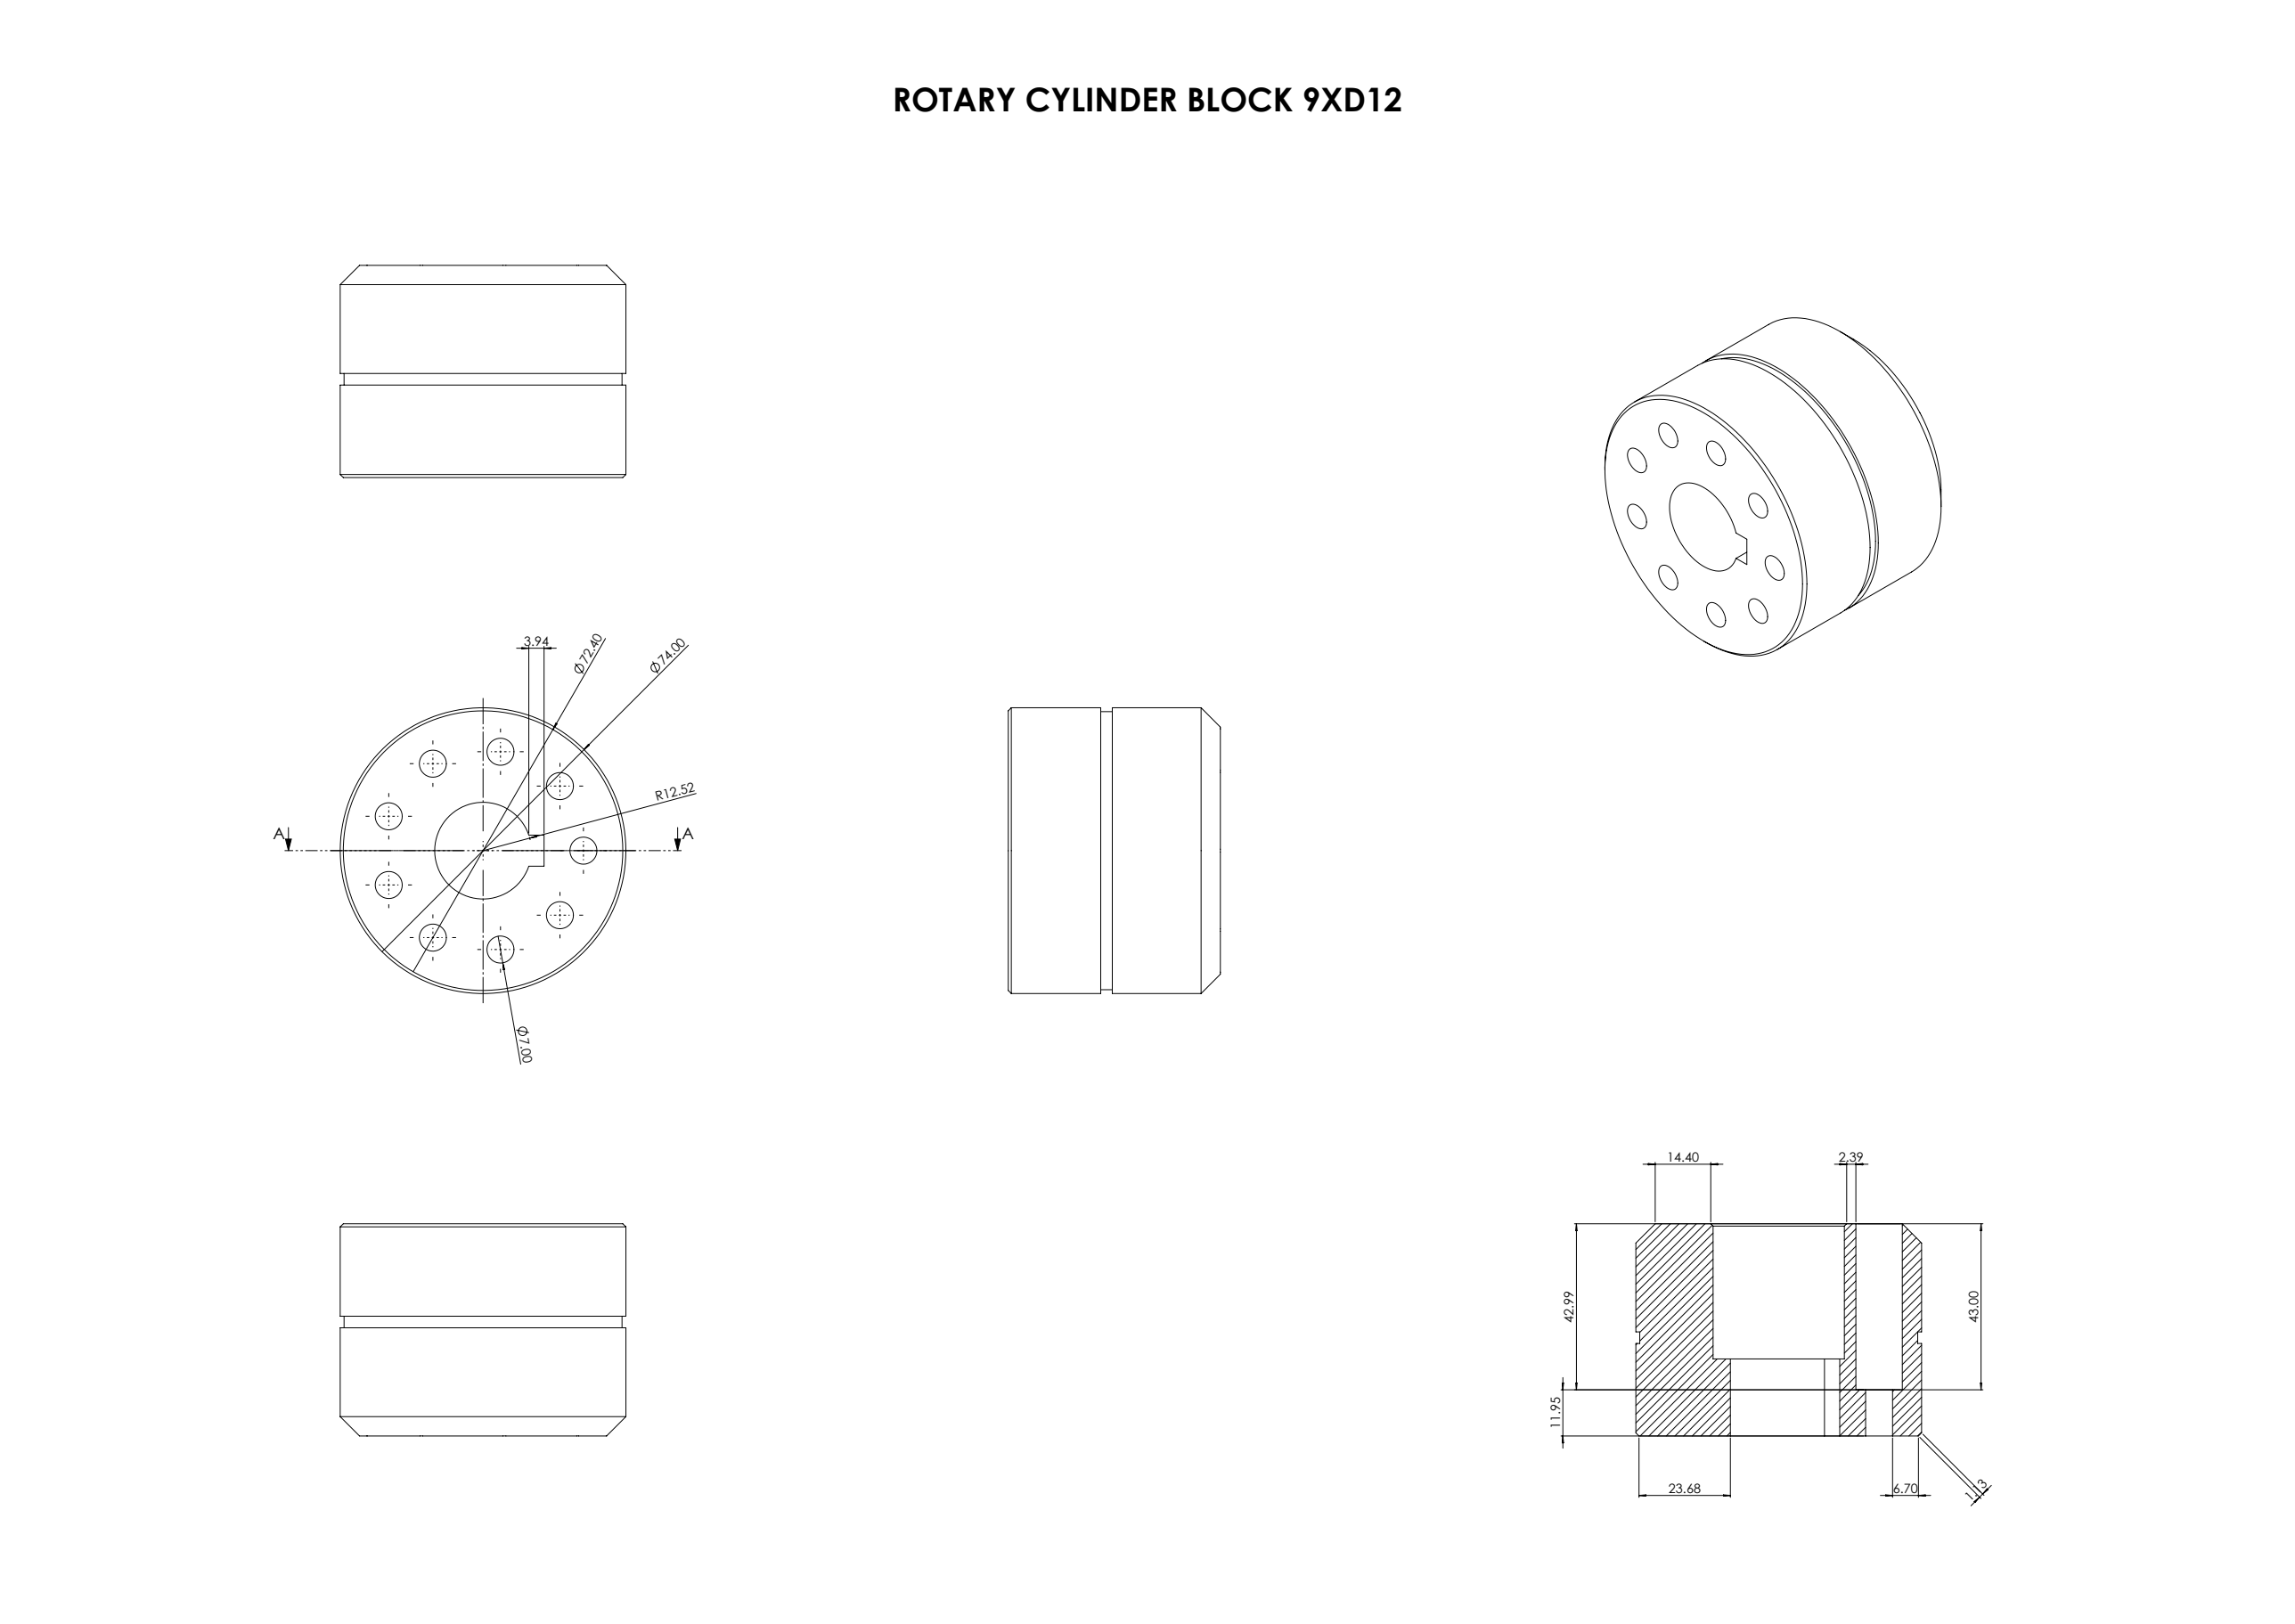
ISO-10303-21;
HEADER;
/* Generated by software containing ST-Developer
 * from STEP Tools, Inc. (www.steptools.com) 
 */

FILE_DESCRIPTION(
/* description */ (''),
/* implementation_level */ '2;1');

FILE_NAME(
/* name */ '05_Rotary_Cylinder_Block_9xD12.step',
/* time_stamp */ '2026-10-23T00:52:27+05:00',
/* author */ (''),
/* organization */ (''),
/* preprocessor_version */ 'ST-DEVELOPER v20.2',
/* originating_system */ 'Autodesk Translation Framework v15.15.0.0',
/* authorisation */ '');

FILE_SCHEMA (('AUTOMOTIVE_DESIGN { 1 0 10303 214 3 1 1 }'));
ENDSEC;

DATA;
#10=MECHANICAL_DESIGN_GEOMETRIC_PRESENTATION_REPRESENTATION('',(#1557),#59204);
#683=B_SPLINE_CURVE_WITH_KNOTS('',3,(#42129,#42130,#42131,#42132,#42133,
#42134),.UNSPECIFIED.,.F.,.F.,(4,2,4),(1.68069680516896,1.71912851411125,
1.75756022305355),.UNSPECIFIED.);
#684=B_SPLINE_CURVE_WITH_KNOTS('',3,(#42145,#42146,#42147,#42148,#42149,
#42150),.UNSPECIFIED.,.F.,.F.,(4,2,4),(1.68069680516896,1.71912851411125,
1.75756022305355),.UNSPECIFIED.);
#685=B_SPLINE_CURVE_WITH_KNOTS('',3,(#42161,#42162,#42163,#42164,#42165,
#42166),.UNSPECIFIED.,.F.,.F.,(4,2,4),(1.68069680516896,1.71912851411125,
1.75756022305355),.UNSPECIFIED.);
#686=B_SPLINE_CURVE_WITH_KNOTS('',3,(#42177,#42178,#42179,#42180,#42181,
#42182),.UNSPECIFIED.,.F.,.F.,(4,2,4),(1.68069680516896,1.71912851411125,
1.75756022305355),.UNSPECIFIED.);
#687=B_SPLINE_CURVE_WITH_KNOTS('',3,(#42193,#42194,#42195,#42196,#42197,
#42198),.UNSPECIFIED.,.F.,.F.,(4,2,4),(1.68069680516897,1.71912851411125,
1.75756022305354),.UNSPECIFIED.);
#688=B_SPLINE_CURVE_WITH_KNOTS('',3,(#42209,#42210,#42211,#42212,#42213,
#42214),.UNSPECIFIED.,.F.,.F.,(4,2,4),(1.68069680516896,1.71912851411125,
1.75756022305355),.UNSPECIFIED.);
#689=B_SPLINE_CURVE_WITH_KNOTS('',3,(#42225,#42226,#42227,#42228,#42229,
#42230),.UNSPECIFIED.,.F.,.F.,(4,2,4),(1.68069680516896,1.71912851411125,
1.75756022305355),.UNSPECIFIED.);
#690=B_SPLINE_CURVE_WITH_KNOTS('',3,(#42241,#42242,#42243,#42244,#42245,
#42246),.UNSPECIFIED.,.F.,.F.,(4,2,4),(1.68069680516896,1.71912851411125,
1.75756022305355),.UNSPECIFIED.);
#691=B_SPLINE_CURVE_WITH_KNOTS('',3,(#42257,#42258,#42259,#42260,#42261,
#42262),.UNSPECIFIED.,.F.,.F.,(4,2,4),(1.68069680516896,1.71912851411125,
1.75756022305355),.UNSPECIFIED.);
#1517=SHAPE_REPRESENTATION_RELATIONSHIP('SRR','None',#59306,#1537);
#1537=ADVANCED_BREP_SHAPE_REPRESENTATION('',(#1584),#59193);
#1557=STYLED_ITEM('',(#59565),#1584);
#1584=MANIFOLD_SOLID_BREP('Cylinder block',#22813);
#1647=FACE_BOUND('',#4356,.T.);
#1648=FACE_BOUND('',#4359,.T.);
#1649=FACE_BOUND('',#4365,.T.);
#1650=FACE_BOUND('',#4377,.T.);
#1651=FACE_BOUND('',#4380,.T.);
#1652=FACE_BOUND('',#4383,.T.);
#1653=FACE_BOUND('',#4386,.T.);
#1654=FACE_BOUND('',#4389,.T.);
#1655=FACE_BOUND('',#4392,.T.);
#1656=FACE_BOUND('',#4395,.T.);
#1657=FACE_BOUND('',#4398,.T.);
#1658=FACE_BOUND('',#4401,.T.);
#1659=FACE_BOUND('',#4403,.T.);
#1660=FACE_BOUND('',#4410,.T.);
#1661=FACE_BOUND('',#4411,.T.);
#1662=FACE_BOUND('',#4412,.T.);
#1663=FACE_BOUND('',#4413,.T.);
#1664=FACE_BOUND('',#4414,.T.);
#1665=FACE_BOUND('',#4415,.T.);
#1666=FACE_BOUND('',#4416,.T.);
#1667=FACE_BOUND('',#4417,.T.);
#1668=FACE_BOUND('',#4418,.T.);
#1669=FACE_BOUND('',#4419,.T.);
#2003=PLANE('',#23610);
#2004=PLANE('',#23615);
#2005=PLANE('',#23619);
#2006=PLANE('',#23620);
#2007=PLANE('',#23621);
#2008=PLANE('',#23622);
#2009=PLANE('',#23656);
#2010=PLANE('',#23661);
#2011=PLANE('',#23666);
#2012=PLANE('',#23671);
#2013=PLANE('',#23676);
#2014=PLANE('',#23681);
#2015=PLANE('',#23686);
#2016=PLANE('',#23691);
#2017=PLANE('',#23696);
#2018=PLANE('',#23697);
#2019=PLANE('',#23717);
#2481=CYLINDRICAL_SURFACE('',#23613,3.6);
#2482=CYLINDRICAL_SURFACE('',#23617,3.7);
#2483=CYLINDRICAL_SURFACE('',#23625,0.35);
#2484=CYLINDRICAL_SURFACE('',#23628,0.35);
#2485=CYLINDRICAL_SURFACE('',#23631,0.35);
#2486=CYLINDRICAL_SURFACE('',#23634,0.35);
#2487=CYLINDRICAL_SURFACE('',#23637,0.35);
#2488=CYLINDRICAL_SURFACE('',#23640,0.35);
#2489=CYLINDRICAL_SURFACE('',#23643,0.35);
#2490=CYLINDRICAL_SURFACE('',#23646,0.35);
#2491=CYLINDRICAL_SURFACE('',#23649,0.35);
#2492=CYLINDRICAL_SURFACE('',#23652,0.601);
#2493=CYLINDRICAL_SURFACE('',#23657,0.601);
#2494=CYLINDRICAL_SURFACE('',#23662,0.601);
#2495=CYLINDRICAL_SURFACE('',#23667,0.601);
#2496=CYLINDRICAL_SURFACE('',#23672,0.601);
#2497=CYLINDRICAL_SURFACE('',#23677,0.601);
#2498=CYLINDRICAL_SURFACE('',#23682,0.601);
#2499=CYLINDRICAL_SURFACE('',#23687,0.601);
#2500=CYLINDRICAL_SURFACE('',#23692,0.601);
#2501=CYLINDRICAL_SURFACE('',#23709,1.7);
#2502=CYLINDRICAL_SURFACE('',#23713,3.7);
#2503=CYLINDRICAL_SURFACE('',#23719,1.252);
#3002=FACE_OUTER_BOUND('',#4355,.T.);
#3003=FACE_OUTER_BOUND('',#4357,.T.);
#3004=FACE_OUTER_BOUND('',#4358,.T.);
#3005=FACE_OUTER_BOUND('',#4360,.T.);
#3006=FACE_OUTER_BOUND('',#4361,.T.);
#3007=FACE_OUTER_BOUND('',#4362,.T.);
#3008=FACE_OUTER_BOUND('',#4363,.T.);
#3009=FACE_OUTER_BOUND('',#4364,.T.);
#3010=FACE_OUTER_BOUND('',#4366,.T.);
#3011=FACE_OUTER_BOUND('',#4367,.T.);
#3012=FACE_OUTER_BOUND('',#4368,.T.);
#3013=FACE_OUTER_BOUND('',#4369,.T.);
#3014=FACE_OUTER_BOUND('',#4370,.T.);
#3015=FACE_OUTER_BOUND('',#4371,.T.);
#3016=FACE_OUTER_BOUND('',#4372,.T.);
#3017=FACE_OUTER_BOUND('',#4373,.T.);
#3018=FACE_OUTER_BOUND('',#4374,.T.);
#3019=FACE_OUTER_BOUND('',#4375,.T.);
#3020=FACE_OUTER_BOUND('',#4376,.T.);
#3021=FACE_OUTER_BOUND('',#4378,.T.);
#3022=FACE_OUTER_BOUND('',#4379,.T.);
#3023=FACE_OUTER_BOUND('',#4381,.T.);
#3024=FACE_OUTER_BOUND('',#4382,.T.);
#3025=FACE_OUTER_BOUND('',#4384,.T.);
#3026=FACE_OUTER_BOUND('',#4385,.T.);
#3027=FACE_OUTER_BOUND('',#4387,.T.);
#3028=FACE_OUTER_BOUND('',#4388,.T.);
#3029=FACE_OUTER_BOUND('',#4390,.T.);
#3030=FACE_OUTER_BOUND('',#4391,.T.);
#3031=FACE_OUTER_BOUND('',#4393,.T.);
#3032=FACE_OUTER_BOUND('',#4394,.T.);
#3033=FACE_OUTER_BOUND('',#4396,.T.);
#3034=FACE_OUTER_BOUND('',#4397,.T.);
#3035=FACE_OUTER_BOUND('',#4399,.T.);
#3036=FACE_OUTER_BOUND('',#4400,.T.);
#3037=FACE_OUTER_BOUND('',#4402,.T.);
#3038=FACE_OUTER_BOUND('',#4404,.T.);
#3039=FACE_OUTER_BOUND('',#4405,.T.);
#3040=FACE_OUTER_BOUND('',#4406,.T.);
#3041=FACE_OUTER_BOUND('',#4407,.T.);
#3042=FACE_OUTER_BOUND('',#4408,.T.);
#3043=FACE_OUTER_BOUND('',#4409,.T.);
#3044=FACE_OUTER_BOUND('',#4420,.T.);
#4355=EDGE_LOOP('',(#16216));
#4356=EDGE_LOOP('',(#16217));
#4357=EDGE_LOOP('',(#16218,#16219,#16220,#16221));
#4358=EDGE_LOOP('',(#16222));
#4359=EDGE_LOOP('',(#16223));
#4360=EDGE_LOOP('',(#16224,#16225,#16226,#16227));
#4361=EDGE_LOOP('',(#16228,#16229,#16230,#16231));
#4362=EDGE_LOOP('',(#16232,#16233,#16234,#16235));
#4363=EDGE_LOOP('',(#16236,#16237,#16238,#16239));
#4364=EDGE_LOOP('',(#16240));
#4365=EDGE_LOOP('',(#16241,#16242,#16243,#16244));
#4366=EDGE_LOOP('',(#16245,#16246,#16247,#16248));
#4367=EDGE_LOOP('',(#16249,#16250,#16251,#16252));
#4368=EDGE_LOOP('',(#16253,#16254,#16255,#16256));
#4369=EDGE_LOOP('',(#16257,#16258,#16259,#16260));
#4370=EDGE_LOOP('',(#16261,#16262,#16263,#16264));
#4371=EDGE_LOOP('',(#16265,#16266,#16267,#16268));
#4372=EDGE_LOOP('',(#16269,#16270,#16271,#16272));
#4373=EDGE_LOOP('',(#16273,#16274,#16275,#16276));
#4374=EDGE_LOOP('',(#16277,#16278,#16279,#16280));
#4375=EDGE_LOOP('',(#16281,#16282,#16283,#16284,#16285,#16286));
#4376=EDGE_LOOP('',(#16287));
#4377=EDGE_LOOP('',(#16288));
#4378=EDGE_LOOP('',(#16289,#16290,#16291,#16292,#16293,#16294));
#4379=EDGE_LOOP('',(#16295));
#4380=EDGE_LOOP('',(#16296));
#4381=EDGE_LOOP('',(#16297,#16298,#16299,#16300,#16301,#16302));
#4382=EDGE_LOOP('',(#16303));
#4383=EDGE_LOOP('',(#16304));
#4384=EDGE_LOOP('',(#16305,#16306,#16307,#16308,#16309,#16310));
#4385=EDGE_LOOP('',(#16311));
#4386=EDGE_LOOP('',(#16312));
#4387=EDGE_LOOP('',(#16313,#16314,#16315,#16316,#16317,#16318));
#4388=EDGE_LOOP('',(#16319));
#4389=EDGE_LOOP('',(#16320));
#4390=EDGE_LOOP('',(#16321,#16322,#16323,#16324,#16325,#16326));
#4391=EDGE_LOOP('',(#16327));
#4392=EDGE_LOOP('',(#16328));
#4393=EDGE_LOOP('',(#16329,#16330,#16331,#16332,#16333,#16334));
#4394=EDGE_LOOP('',(#16335));
#4395=EDGE_LOOP('',(#16336));
#4396=EDGE_LOOP('',(#16337,#16338,#16339,#16340,#16341,#16342));
#4397=EDGE_LOOP('',(#16343));
#4398=EDGE_LOOP('',(#16344));
#4399=EDGE_LOOP('',(#16345,#16346,#16347,#16348,#16349,#16350));
#4400=EDGE_LOOP('',(#16351));
#4401=EDGE_LOOP('',(#16352));
#4402=EDGE_LOOP('',(#16353,#16354,#16355,#16356,#16357,#16358,#16359,#16360,
#16361,#16362,#16363,#16364,#16365,#16366,#16367,#16368,#16369,#16370,#16371,
#16372,#16373,#16374,#16375,#16376,#16377,#16378,#16379,#16380));
#4403=EDGE_LOOP('',(#16381));
#4404=EDGE_LOOP('',(#16382,#16383,#16384,#16385));
#4405=EDGE_LOOP('',(#16386,#16387,#16388,#16389));
#4406=EDGE_LOOP('',(#16390,#16391,#16392,#16393,#16394,#16395,#16396,#16397,
#16398,#16399,#16400,#16401,#16402,#16403,#16404,#16405,#16406,#16407,#16408,
#16409,#16410,#16411));
#4407=EDGE_LOOP('',(#16412,#16413,#16414,#16415));
#4408=EDGE_LOOP('',(#16416,#16417,#16418,#16419));
#4409=EDGE_LOOP('',(#16420));
#4410=EDGE_LOOP('',(#16421));
#4411=EDGE_LOOP('',(#16422));
#4412=EDGE_LOOP('',(#16423));
#4413=EDGE_LOOP('',(#16424));
#4414=EDGE_LOOP('',(#16425));
#4415=EDGE_LOOP('',(#16426));
#4416=EDGE_LOOP('',(#16427));
#4417=EDGE_LOOP('',(#16428));
#4418=EDGE_LOOP('',(#16429));
#4419=EDGE_LOOP('',(#16430,#16431,#16432,#16433));
#4420=EDGE_LOOP('',(#16434,#16435,#16436,#16437));
#5884=LINE('',#42039,#7317);
#5885=LINE('',#42045,#7318);
#5886=LINE('',#42050,#7319);
#5887=LINE('',#42052,#7320);
#5888=LINE('',#42054,#7321);
#5889=LINE('',#42055,#7322);
#5890=LINE('',#42058,#7323);
#5891=LINE('',#42060,#7324);
#5892=LINE('',#42061,#7325);
#5893=LINE('',#42065,#7326);
#5894=LINE('',#42066,#7327);
#5895=LINE('',#42067,#7328);
#5896=LINE('',#42076,#7329);
#5897=LINE('',#42082,#7330);
#5898=LINE('',#42088,#7331);
#5899=LINE('',#42094,#7332);
#5900=LINE('',#42100,#7333);
#5901=LINE('',#42106,#7334);
#5902=LINE('',#42112,#7335);
#5903=LINE('',#42118,#7336);
#5904=LINE('',#42124,#7337);
#5905=LINE('',#42138,#7338);
#5906=LINE('',#42154,#7339);
#5907=LINE('',#42170,#7340);
#5908=LINE('',#42186,#7341);
#5909=LINE('',#42202,#7342);
#5910=LINE('',#42218,#7343);
#5911=LINE('',#42234,#7344);
#5912=LINE('',#42250,#7345);
#5913=LINE('',#42266,#7346);
#5914=LINE('',#42286,#7347);
#5915=LINE('',#42289,#7348);
#5916=LINE('',#42291,#7349);
#5917=LINE('',#42295,#7350);
#5918=LINE('',#42299,#7351);
#7317=VECTOR('',#26650,3.6);
#7318=VECTOR('',#26657,3.7);
#7319=VECTOR('',#26662,1.);
#7320=VECTOR('',#26663,1.);
#7321=VECTOR('',#26664,1.);
#7322=VECTOR('',#26665,1.);
#7323=VECTOR('',#26668,1.);
#7324=VECTOR('',#26669,1.);
#7325=VECTOR('',#26670,1.);
#7326=VECTOR('',#26673,1.);
#7327=VECTOR('',#26674,1.);
#7328=VECTOR('',#26675,1.);
#7329=VECTOR('',#26686,0.35);
#7330=VECTOR('',#26693,0.35);
#7331=VECTOR('',#26700,0.35);
#7332=VECTOR('',#26707,0.35);
#7333=VECTOR('',#26714,0.35);
#7334=VECTOR('',#26721,0.35);
#7335=VECTOR('',#26728,0.35);
#7336=VECTOR('',#26735,0.35);
#7337=VECTOR('',#26742,0.35);
#7338=VECTOR('',#26749,0.601);
#7339=VECTOR('',#26760,0.601);
#7340=VECTOR('',#26771,0.601);
#7341=VECTOR('',#26782,0.601);
#7342=VECTOR('',#26793,0.601);
#7343=VECTOR('',#26804,0.601);
#7344=VECTOR('',#26815,0.601);
#7345=VECTOR('',#26826,0.601);
#7346=VECTOR('',#26837,0.601);
#7347=VECTOR('',#26870,1.7);
#7348=VECTOR('',#26875,1.73);
#7349=VECTOR('',#26878,3.45);
#7350=VECTOR('',#26883,3.7);
#7351=VECTOR('',#26888,3.66);
#8595=CIRCLE('',#23611,3.7);
#8596=CIRCLE('',#23612,3.6);
#8597=CIRCLE('',#23614,3.6);
#8598=CIRCLE('',#23616,3.7);
#8599=CIRCLE('',#23618,3.7);
#8600=CIRCLE('',#23623,1.7);
#8601=CIRCLE('',#23624,1.252);
#8602=CIRCLE('',#23626,0.35);
#8603=CIRCLE('',#23627,0.35);
#8604=CIRCLE('',#23629,0.35);
#8605=CIRCLE('',#23630,0.35);
#8606=CIRCLE('',#23632,0.35);
#8607=CIRCLE('',#23633,0.35);
#8608=CIRCLE('',#23635,0.35);
#8609=CIRCLE('',#23636,0.35);
#8610=CIRCLE('',#23638,0.35);
#8611=CIRCLE('',#23639,0.35);
#8612=CIRCLE('',#23641,0.35);
#8613=CIRCLE('',#23642,0.35);
#8614=CIRCLE('',#23644,0.35);
#8615=CIRCLE('',#23645,0.35);
#8616=CIRCLE('',#23647,0.35);
#8617=CIRCLE('',#23648,0.35);
#8618=CIRCLE('',#23650,0.35);
#8619=CIRCLE('',#23651,0.35);
#8620=CIRCLE('',#23653,0.601);
#8621=CIRCLE('',#23654,0.601);
#8622=CIRCLE('',#23655,0.601);
#8623=CIRCLE('',#23658,0.601);
#8624=CIRCLE('',#23659,0.601);
#8625=CIRCLE('',#23660,0.601);
#8626=CIRCLE('',#23663,0.601);
#8627=CIRCLE('',#23664,0.601);
#8628=CIRCLE('',#23665,0.601);
#8629=CIRCLE('',#23668,0.601);
#8630=CIRCLE('',#23669,0.601);
#8631=CIRCLE('',#23670,0.601);
#8632=CIRCLE('',#23673,0.601);
#8633=CIRCLE('',#23674,0.601);
#8634=CIRCLE('',#23675,0.601);
#8635=CIRCLE('',#23678,0.601);
#8636=CIRCLE('',#23679,0.601);
#8637=CIRCLE('',#23680,0.601);
#8638=CIRCLE('',#23683,0.601);
#8639=CIRCLE('',#23684,0.601);
#8640=CIRCLE('',#23685,0.601);
#8641=CIRCLE('',#23688,0.601);
#8642=CIRCLE('',#23689,0.601);
#8643=CIRCLE('',#23690,0.601);
#8644=CIRCLE('',#23693,0.601);
#8645=CIRCLE('',#23694,0.601);
#8646=CIRCLE('',#23695,0.601);
#8647=CIRCLE('',#23698,3.2);
#8648=CIRCLE('',#23699,3.2);
#8649=CIRCLE('',#23700,3.2);
#8650=CIRCLE('',#23701,3.2);
#8651=CIRCLE('',#23702,3.2);
#8652=CIRCLE('',#23703,3.2);
#8653=CIRCLE('',#23704,3.2);
#8654=CIRCLE('',#23705,3.2);
#8655=CIRCLE('',#23706,3.2);
#8656=CIRCLE('',#23707,3.2);
#8657=CIRCLE('',#23708,1.76);
#8658=CIRCLE('',#23710,1.7);
#8659=CIRCLE('',#23714,3.7);
#8660=CIRCLE('',#23716,3.62);
#8661=CIRCLE('',#23718,1.252);
#9676=VERTEX_POINT('',#42032);
#9677=VERTEX_POINT('',#42034);
#9678=VERTEX_POINT('',#42037);
#9679=VERTEX_POINT('',#42041);
#9680=VERTEX_POINT('',#42044);
#9681=VERTEX_POINT('',#42048);
#9682=VERTEX_POINT('',#42049);
#9683=VERTEX_POINT('',#42051);
#9684=VERTEX_POINT('',#42053);
#9685=VERTEX_POINT('',#42057);
#9686=VERTEX_POINT('',#42059);
#9687=VERTEX_POINT('',#42063);
#9688=VERTEX_POINT('',#42064);
#9689=VERTEX_POINT('',#42069);
#9690=VERTEX_POINT('',#42073);
#9691=VERTEX_POINT('',#42075);
#9692=VERTEX_POINT('',#42079);
#9693=VERTEX_POINT('',#42081);
#9694=VERTEX_POINT('',#42085);
#9695=VERTEX_POINT('',#42087);
#9696=VERTEX_POINT('',#42091);
#9697=VERTEX_POINT('',#42093);
#9698=VERTEX_POINT('',#42097);
#9699=VERTEX_POINT('',#42099);
#9700=VERTEX_POINT('',#42103);
#9701=VERTEX_POINT('',#42105);
#9702=VERTEX_POINT('',#42109);
#9703=VERTEX_POINT('',#42111);
#9704=VERTEX_POINT('',#42115);
#9705=VERTEX_POINT('',#42117);
#9706=VERTEX_POINT('',#42121);
#9707=VERTEX_POINT('',#42123);
#9708=VERTEX_POINT('',#42127);
#9709=VERTEX_POINT('',#42128);
#9710=VERTEX_POINT('',#42135);
#9711=VERTEX_POINT('',#42137);
#9712=VERTEX_POINT('',#42143);
#9713=VERTEX_POINT('',#42144);
#9714=VERTEX_POINT('',#42151);
#9715=VERTEX_POINT('',#42153);
#9716=VERTEX_POINT('',#42159);
#9717=VERTEX_POINT('',#42160);
#9718=VERTEX_POINT('',#42167);
#9719=VERTEX_POINT('',#42169);
#9720=VERTEX_POINT('',#42175);
#9721=VERTEX_POINT('',#42176);
#9722=VERTEX_POINT('',#42183);
#9723=VERTEX_POINT('',#42185);
#9724=VERTEX_POINT('',#42191);
#9725=VERTEX_POINT('',#42192);
#9726=VERTEX_POINT('',#42199);
#9727=VERTEX_POINT('',#42201);
#9728=VERTEX_POINT('',#42207);
#9729=VERTEX_POINT('',#42208);
#9730=VERTEX_POINT('',#42215);
#9731=VERTEX_POINT('',#42217);
#9732=VERTEX_POINT('',#42223);
#9733=VERTEX_POINT('',#42224);
#9734=VERTEX_POINT('',#42231);
#9735=VERTEX_POINT('',#42233);
#9736=VERTEX_POINT('',#42239);
#9737=VERTEX_POINT('',#42240);
#9738=VERTEX_POINT('',#42247);
#9739=VERTEX_POINT('',#42249);
#9740=VERTEX_POINT('',#42255);
#9741=VERTEX_POINT('',#42256);
#9742=VERTEX_POINT('',#42263);
#9743=VERTEX_POINT('',#42265);
#9744=VERTEX_POINT('',#42273);
#9745=VERTEX_POINT('',#42282);
#9746=VERTEX_POINT('',#42285);
#9747=VERTEX_POINT('',#42293);
#9748=VERTEX_POINT('',#42297);
#12112=EDGE_CURVE('',#9676,#9676,#8595,.T.);
#12113=EDGE_CURVE('',#9677,#9677,#8596,.T.);
#12114=EDGE_CURVE('',#9678,#9678,#8597,.T.);
#12115=EDGE_CURVE('',#9678,#9677,#5884,.T.);
#12116=EDGE_CURVE('',#9679,#9679,#8598,.T.);
#12117=EDGE_CURVE('',#9679,#9680,#5885,.T.);
#12118=EDGE_CURVE('',#9680,#9680,#8599,.T.);
#12119=EDGE_CURVE('',#9681,#9682,#5886,.T.);
#12120=EDGE_CURVE('',#9683,#9681,#5887,.T.);
#12121=EDGE_CURVE('',#9683,#9684,#5888,.T.);
#12122=EDGE_CURVE('',#9682,#9684,#5889,.T.);
#12123=EDGE_CURVE('',#9684,#9685,#5890,.T.);
#12124=EDGE_CURVE('',#9686,#9683,#5891,.T.);
#12125=EDGE_CURVE('',#9686,#9685,#5892,.T.);
#12126=EDGE_CURVE('',#9687,#9688,#5893,.T.);
#12127=EDGE_CURVE('',#9685,#9687,#5894,.T.);
#12128=EDGE_CURVE('',#9688,#9686,#5895,.T.);
#12129=EDGE_CURVE('',#9689,#9689,#8600,.T.);
#12130=EDGE_CURVE('',#9681,#9688,#8601,.T.);
#12131=EDGE_CURVE('',#9690,#9690,#8602,.T.);
#12132=EDGE_CURVE('',#9690,#9691,#5896,.T.);
#12133=EDGE_CURVE('',#9691,#9691,#8603,.T.);
#12134=EDGE_CURVE('',#9692,#9692,#8604,.T.);
#12135=EDGE_CURVE('',#9692,#9693,#5897,.T.);
#12136=EDGE_CURVE('',#9693,#9693,#8605,.T.);
#12137=EDGE_CURVE('',#9694,#9694,#8606,.T.);
#12138=EDGE_CURVE('',#9694,#9695,#5898,.T.);
#12139=EDGE_CURVE('',#9695,#9695,#8607,.T.);
#12140=EDGE_CURVE('',#9696,#9696,#8608,.T.);
#12141=EDGE_CURVE('',#9696,#9697,#5899,.T.);
#12142=EDGE_CURVE('',#9697,#9697,#8609,.T.);
#12143=EDGE_CURVE('',#9698,#9698,#8610,.T.);
#12144=EDGE_CURVE('',#9698,#9699,#5900,.T.);
#12145=EDGE_CURVE('',#9699,#9699,#8611,.T.);
#12146=EDGE_CURVE('',#9700,#9700,#8612,.T.);
#12147=EDGE_CURVE('',#9700,#9701,#5901,.T.);
#12148=EDGE_CURVE('',#9701,#9701,#8613,.T.);
#12149=EDGE_CURVE('',#9702,#9702,#8614,.T.);
#12150=EDGE_CURVE('',#9702,#9703,#5902,.T.);
#12151=EDGE_CURVE('',#9703,#9703,#8615,.T.);
#12152=EDGE_CURVE('',#9704,#9704,#8616,.T.);
#12153=EDGE_CURVE('',#9704,#9705,#5903,.T.);
#12154=EDGE_CURVE('',#9705,#9705,#8617,.T.);
#12155=EDGE_CURVE('',#9706,#9706,#8618,.T.);
#12156=EDGE_CURVE('',#9706,#9707,#5904,.T.);
#12157=EDGE_CURVE('',#9707,#9707,#8619,.T.);
#12158=EDGE_CURVE('',#9708,#9709,#683,.T.);
#12159=EDGE_CURVE('',#9710,#9708,#8620,.T.);
#12160=EDGE_CURVE('',#9710,#9711,#5905,.T.);
#12161=EDGE_CURVE('',#9711,#9711,#8621,.T.);
#12162=EDGE_CURVE('',#9709,#9710,#8622,.T.);
#12163=EDGE_CURVE('',#9712,#9713,#684,.T.);
#12164=EDGE_CURVE('',#9714,#9712,#8623,.T.);
#12165=EDGE_CURVE('',#9714,#9715,#5906,.T.);
#12166=EDGE_CURVE('',#9715,#9715,#8624,.T.);
#12167=EDGE_CURVE('',#9713,#9714,#8625,.T.);
#12168=EDGE_CURVE('',#9716,#9717,#685,.T.);
#12169=EDGE_CURVE('',#9718,#9716,#8626,.T.);
#12170=EDGE_CURVE('',#9718,#9719,#5907,.T.);
#12171=EDGE_CURVE('',#9719,#9719,#8627,.T.);
#12172=EDGE_CURVE('',#9717,#9718,#8628,.T.);
#12173=EDGE_CURVE('',#9720,#9721,#686,.T.);
#12174=EDGE_CURVE('',#9722,#9720,#8629,.T.);
#12175=EDGE_CURVE('',#9722,#9723,#5908,.T.);
#12176=EDGE_CURVE('',#9723,#9723,#8630,.T.);
#12177=EDGE_CURVE('',#9721,#9722,#8631,.T.);
#12178=EDGE_CURVE('',#9724,#9725,#687,.T.);
#12179=EDGE_CURVE('',#9726,#9724,#8632,.T.);
#12180=EDGE_CURVE('',#9726,#9727,#5909,.T.);
#12181=EDGE_CURVE('',#9727,#9727,#8633,.T.);
#12182=EDGE_CURVE('',#9725,#9726,#8634,.T.);
#12183=EDGE_CURVE('',#9728,#9729,#688,.T.);
#12184=EDGE_CURVE('',#9730,#9728,#8635,.T.);
#12185=EDGE_CURVE('',#9730,#9731,#5910,.T.);
#12186=EDGE_CURVE('',#9731,#9731,#8636,.T.);
#12187=EDGE_CURVE('',#9729,#9730,#8637,.T.);
#12188=EDGE_CURVE('',#9732,#9733,#689,.T.);
#12189=EDGE_CURVE('',#9734,#9732,#8638,.T.);
#12190=EDGE_CURVE('',#9734,#9735,#5911,.T.);
#12191=EDGE_CURVE('',#9735,#9735,#8639,.T.);
#12192=EDGE_CURVE('',#9733,#9734,#8640,.T.);
#12193=EDGE_CURVE('',#9736,#9737,#690,.T.);
#12194=EDGE_CURVE('',#9738,#9736,#8641,.T.);
#12195=EDGE_CURVE('',#9738,#9739,#5912,.T.);
#12196=EDGE_CURVE('',#9739,#9739,#8642,.T.);
#12197=EDGE_CURVE('',#9737,#9738,#8643,.T.);
#12198=EDGE_CURVE('',#9740,#9741,#691,.T.);
#12199=EDGE_CURVE('',#9742,#9740,#8644,.T.);
#12200=EDGE_CURVE('',#9742,#9743,#5913,.T.);
#12201=EDGE_CURVE('',#9743,#9743,#8645,.T.);
#12202=EDGE_CURVE('',#9741,#9742,#8646,.T.);
#12203=EDGE_CURVE('',#9737,#9708,#8647,.T.);
#12204=EDGE_CURVE('',#9713,#9736,#8648,.T.);
#12205=EDGE_CURVE('',#9744,#9712,#8649,.T.);
#12206=EDGE_CURVE('',#9717,#9744,#8650,.T.);
#12207=EDGE_CURVE('',#9729,#9716,#8651,.T.);
#12208=EDGE_CURVE('',#9721,#9728,#8652,.T.);
#12209=EDGE_CURVE('',#9725,#9720,#8653,.T.);
#12210=EDGE_CURVE('',#9733,#9724,#8654,.T.);
#12211=EDGE_CURVE('',#9741,#9732,#8655,.T.);
#12212=EDGE_CURVE('',#9709,#9740,#8656,.T.);
#12213=EDGE_CURVE('',#9745,#9745,#8657,.T.);
#12214=EDGE_CURVE('',#9689,#9746,#5914,.T.);
#12215=EDGE_CURVE('',#9746,#9746,#8658,.T.);
#12216=EDGE_CURVE('',#9746,#9745,#5915,.T.);
#12217=EDGE_CURVE('',#9680,#9744,#5916,.T.);
#12218=EDGE_CURVE('',#9747,#9747,#8659,.T.);
#12219=EDGE_CURVE('',#9747,#9676,#5917,.T.);
#12220=EDGE_CURVE('',#9748,#9748,#8660,.T.);
#12221=EDGE_CURVE('',#9748,#9747,#5918,.T.);
#12222=EDGE_CURVE('',#9682,#9687,#8661,.T.);
#16216=ORIENTED_EDGE('',*,*,#12112,.F.);
#16217=ORIENTED_EDGE('',*,*,#12113,.T.);
#16218=ORIENTED_EDGE('',*,*,#12114,.T.);
#16219=ORIENTED_EDGE('',*,*,#12115,.T.);
#16220=ORIENTED_EDGE('',*,*,#12113,.F.);
#16221=ORIENTED_EDGE('',*,*,#12115,.F.);
#16222=ORIENTED_EDGE('',*,*,#12116,.F.);
#16223=ORIENTED_EDGE('',*,*,#12114,.F.);
#16224=ORIENTED_EDGE('',*,*,#12116,.T.);
#16225=ORIENTED_EDGE('',*,*,#12117,.T.);
#16226=ORIENTED_EDGE('',*,*,#12118,.T.);
#16227=ORIENTED_EDGE('',*,*,#12117,.F.);
#16228=ORIENTED_EDGE('',*,*,#12119,.F.);
#16229=ORIENTED_EDGE('',*,*,#12120,.F.);
#16230=ORIENTED_EDGE('',*,*,#12121,.T.);
#16231=ORIENTED_EDGE('',*,*,#12122,.F.);
#16232=ORIENTED_EDGE('',*,*,#12123,.F.);
#16233=ORIENTED_EDGE('',*,*,#12121,.F.);
#16234=ORIENTED_EDGE('',*,*,#12124,.F.);
#16235=ORIENTED_EDGE('',*,*,#12125,.T.);
#16236=ORIENTED_EDGE('',*,*,#12126,.F.);
#16237=ORIENTED_EDGE('',*,*,#12127,.F.);
#16238=ORIENTED_EDGE('',*,*,#12125,.F.);
#16239=ORIENTED_EDGE('',*,*,#12128,.F.);
#16240=ORIENTED_EDGE('',*,*,#12129,.F.);
#16241=ORIENTED_EDGE('',*,*,#12128,.T.);
#16242=ORIENTED_EDGE('',*,*,#12124,.T.);
#16243=ORIENTED_EDGE('',*,*,#12120,.T.);
#16244=ORIENTED_EDGE('',*,*,#12130,.T.);
#16245=ORIENTED_EDGE('',*,*,#12131,.F.);
#16246=ORIENTED_EDGE('',*,*,#12132,.T.);
#16247=ORIENTED_EDGE('',*,*,#12133,.F.);
#16248=ORIENTED_EDGE('',*,*,#12132,.F.);
#16249=ORIENTED_EDGE('',*,*,#12134,.F.);
#16250=ORIENTED_EDGE('',*,*,#12135,.T.);
#16251=ORIENTED_EDGE('',*,*,#12136,.F.);
#16252=ORIENTED_EDGE('',*,*,#12135,.F.);
#16253=ORIENTED_EDGE('',*,*,#12137,.F.);
#16254=ORIENTED_EDGE('',*,*,#12138,.T.);
#16255=ORIENTED_EDGE('',*,*,#12139,.F.);
#16256=ORIENTED_EDGE('',*,*,#12138,.F.);
#16257=ORIENTED_EDGE('',*,*,#12140,.F.);
#16258=ORIENTED_EDGE('',*,*,#12141,.T.);
#16259=ORIENTED_EDGE('',*,*,#12142,.F.);
#16260=ORIENTED_EDGE('',*,*,#12141,.F.);
#16261=ORIENTED_EDGE('',*,*,#12143,.F.);
#16262=ORIENTED_EDGE('',*,*,#12144,.T.);
#16263=ORIENTED_EDGE('',*,*,#12145,.F.);
#16264=ORIENTED_EDGE('',*,*,#12144,.F.);
#16265=ORIENTED_EDGE('',*,*,#12146,.F.);
#16266=ORIENTED_EDGE('',*,*,#12147,.T.);
#16267=ORIENTED_EDGE('',*,*,#12148,.F.);
#16268=ORIENTED_EDGE('',*,*,#12147,.F.);
#16269=ORIENTED_EDGE('',*,*,#12149,.F.);
#16270=ORIENTED_EDGE('',*,*,#12150,.T.);
#16271=ORIENTED_EDGE('',*,*,#12151,.F.);
#16272=ORIENTED_EDGE('',*,*,#12150,.F.);
#16273=ORIENTED_EDGE('',*,*,#12152,.F.);
#16274=ORIENTED_EDGE('',*,*,#12153,.T.);
#16275=ORIENTED_EDGE('',*,*,#12154,.F.);
#16276=ORIENTED_EDGE('',*,*,#12153,.F.);
#16277=ORIENTED_EDGE('',*,*,#12155,.F.);
#16278=ORIENTED_EDGE('',*,*,#12156,.T.);
#16279=ORIENTED_EDGE('',*,*,#12157,.F.);
#16280=ORIENTED_EDGE('',*,*,#12156,.F.);
#16281=ORIENTED_EDGE('',*,*,#12158,.F.);
#16282=ORIENTED_EDGE('',*,*,#12159,.F.);
#16283=ORIENTED_EDGE('',*,*,#12160,.T.);
#16284=ORIENTED_EDGE('',*,*,#12161,.T.);
#16285=ORIENTED_EDGE('',*,*,#12160,.F.);
#16286=ORIENTED_EDGE('',*,*,#12162,.F.);
#16287=ORIENTED_EDGE('',*,*,#12161,.F.);
#16288=ORIENTED_EDGE('',*,*,#12131,.T.);
#16289=ORIENTED_EDGE('',*,*,#12163,.F.);
#16290=ORIENTED_EDGE('',*,*,#12164,.F.);
#16291=ORIENTED_EDGE('',*,*,#12165,.T.);
#16292=ORIENTED_EDGE('',*,*,#12166,.T.);
#16293=ORIENTED_EDGE('',*,*,#12165,.F.);
#16294=ORIENTED_EDGE('',*,*,#12167,.F.);
#16295=ORIENTED_EDGE('',*,*,#12166,.F.);
#16296=ORIENTED_EDGE('',*,*,#12134,.T.);
#16297=ORIENTED_EDGE('',*,*,#12168,.F.);
#16298=ORIENTED_EDGE('',*,*,#12169,.F.);
#16299=ORIENTED_EDGE('',*,*,#12170,.T.);
#16300=ORIENTED_EDGE('',*,*,#12171,.T.);
#16301=ORIENTED_EDGE('',*,*,#12170,.F.);
#16302=ORIENTED_EDGE('',*,*,#12172,.F.);
#16303=ORIENTED_EDGE('',*,*,#12171,.F.);
#16304=ORIENTED_EDGE('',*,*,#12137,.T.);
#16305=ORIENTED_EDGE('',*,*,#12173,.F.);
#16306=ORIENTED_EDGE('',*,*,#12174,.F.);
#16307=ORIENTED_EDGE('',*,*,#12175,.T.);
#16308=ORIENTED_EDGE('',*,*,#12176,.T.);
#16309=ORIENTED_EDGE('',*,*,#12175,.F.);
#16310=ORIENTED_EDGE('',*,*,#12177,.F.);
#16311=ORIENTED_EDGE('',*,*,#12176,.F.);
#16312=ORIENTED_EDGE('',*,*,#12140,.T.);
#16313=ORIENTED_EDGE('',*,*,#12178,.F.);
#16314=ORIENTED_EDGE('',*,*,#12179,.F.);
#16315=ORIENTED_EDGE('',*,*,#12180,.T.);
#16316=ORIENTED_EDGE('',*,*,#12181,.T.);
#16317=ORIENTED_EDGE('',*,*,#12180,.F.);
#16318=ORIENTED_EDGE('',*,*,#12182,.F.);
#16319=ORIENTED_EDGE('',*,*,#12181,.F.);
#16320=ORIENTED_EDGE('',*,*,#12143,.T.);
#16321=ORIENTED_EDGE('',*,*,#12183,.F.);
#16322=ORIENTED_EDGE('',*,*,#12184,.F.);
#16323=ORIENTED_EDGE('',*,*,#12185,.T.);
#16324=ORIENTED_EDGE('',*,*,#12186,.T.);
#16325=ORIENTED_EDGE('',*,*,#12185,.F.);
#16326=ORIENTED_EDGE('',*,*,#12187,.F.);
#16327=ORIENTED_EDGE('',*,*,#12186,.F.);
#16328=ORIENTED_EDGE('',*,*,#12146,.T.);
#16329=ORIENTED_EDGE('',*,*,#12188,.F.);
#16330=ORIENTED_EDGE('',*,*,#12189,.F.);
#16331=ORIENTED_EDGE('',*,*,#12190,.T.);
#16332=ORIENTED_EDGE('',*,*,#12191,.T.);
#16333=ORIENTED_EDGE('',*,*,#12190,.F.);
#16334=ORIENTED_EDGE('',*,*,#12192,.F.);
#16335=ORIENTED_EDGE('',*,*,#12191,.F.);
#16336=ORIENTED_EDGE('',*,*,#12149,.T.);
#16337=ORIENTED_EDGE('',*,*,#12193,.F.);
#16338=ORIENTED_EDGE('',*,*,#12194,.F.);
#16339=ORIENTED_EDGE('',*,*,#12195,.T.);
#16340=ORIENTED_EDGE('',*,*,#12196,.T.);
#16341=ORIENTED_EDGE('',*,*,#12195,.F.);
#16342=ORIENTED_EDGE('',*,*,#12197,.F.);
#16343=ORIENTED_EDGE('',*,*,#12196,.F.);
#16344=ORIENTED_EDGE('',*,*,#12152,.T.);
#16345=ORIENTED_EDGE('',*,*,#12198,.F.);
#16346=ORIENTED_EDGE('',*,*,#12199,.F.);
#16347=ORIENTED_EDGE('',*,*,#12200,.T.);
#16348=ORIENTED_EDGE('',*,*,#12201,.T.);
#16349=ORIENTED_EDGE('',*,*,#12200,.F.);
#16350=ORIENTED_EDGE('',*,*,#12202,.F.);
#16351=ORIENTED_EDGE('',*,*,#12201,.F.);
#16352=ORIENTED_EDGE('',*,*,#12155,.T.);
#16353=ORIENTED_EDGE('',*,*,#12162,.T.);
#16354=ORIENTED_EDGE('',*,*,#12159,.T.);
#16355=ORIENTED_EDGE('',*,*,#12203,.F.);
#16356=ORIENTED_EDGE('',*,*,#12197,.T.);
#16357=ORIENTED_EDGE('',*,*,#12194,.T.);
#16358=ORIENTED_EDGE('',*,*,#12204,.F.);
#16359=ORIENTED_EDGE('',*,*,#12167,.T.);
#16360=ORIENTED_EDGE('',*,*,#12164,.T.);
#16361=ORIENTED_EDGE('',*,*,#12205,.F.);
#16362=ORIENTED_EDGE('',*,*,#12206,.F.);
#16363=ORIENTED_EDGE('',*,*,#12172,.T.);
#16364=ORIENTED_EDGE('',*,*,#12169,.T.);
#16365=ORIENTED_EDGE('',*,*,#12207,.F.);
#16366=ORIENTED_EDGE('',*,*,#12187,.T.);
#16367=ORIENTED_EDGE('',*,*,#12184,.T.);
#16368=ORIENTED_EDGE('',*,*,#12208,.F.);
#16369=ORIENTED_EDGE('',*,*,#12177,.T.);
#16370=ORIENTED_EDGE('',*,*,#12174,.T.);
#16371=ORIENTED_EDGE('',*,*,#12209,.F.);
#16372=ORIENTED_EDGE('',*,*,#12182,.T.);
#16373=ORIENTED_EDGE('',*,*,#12179,.T.);
#16374=ORIENTED_EDGE('',*,*,#12210,.F.);
#16375=ORIENTED_EDGE('',*,*,#12192,.T.);
#16376=ORIENTED_EDGE('',*,*,#12189,.T.);
#16377=ORIENTED_EDGE('',*,*,#12211,.F.);
#16378=ORIENTED_EDGE('',*,*,#12202,.T.);
#16379=ORIENTED_EDGE('',*,*,#12199,.T.);
#16380=ORIENTED_EDGE('',*,*,#12212,.F.);
#16381=ORIENTED_EDGE('',*,*,#12213,.T.);
#16382=ORIENTED_EDGE('',*,*,#12129,.T.);
#16383=ORIENTED_EDGE('',*,*,#12214,.T.);
#16384=ORIENTED_EDGE('',*,*,#12215,.F.);
#16385=ORIENTED_EDGE('',*,*,#12214,.F.);
#16386=ORIENTED_EDGE('',*,*,#12215,.T.);
#16387=ORIENTED_EDGE('',*,*,#12216,.T.);
#16388=ORIENTED_EDGE('',*,*,#12213,.F.);
#16389=ORIENTED_EDGE('',*,*,#12216,.F.);
#16390=ORIENTED_EDGE('',*,*,#12118,.F.);
#16391=ORIENTED_EDGE('',*,*,#12217,.T.);
#16392=ORIENTED_EDGE('',*,*,#12205,.T.);
#16393=ORIENTED_EDGE('',*,*,#12163,.T.);
#16394=ORIENTED_EDGE('',*,*,#12204,.T.);
#16395=ORIENTED_EDGE('',*,*,#12193,.T.);
#16396=ORIENTED_EDGE('',*,*,#12203,.T.);
#16397=ORIENTED_EDGE('',*,*,#12158,.T.);
#16398=ORIENTED_EDGE('',*,*,#12212,.T.);
#16399=ORIENTED_EDGE('',*,*,#12198,.T.);
#16400=ORIENTED_EDGE('',*,*,#12211,.T.);
#16401=ORIENTED_EDGE('',*,*,#12188,.T.);
#16402=ORIENTED_EDGE('',*,*,#12210,.T.);
#16403=ORIENTED_EDGE('',*,*,#12178,.T.);
#16404=ORIENTED_EDGE('',*,*,#12209,.T.);
#16405=ORIENTED_EDGE('',*,*,#12173,.T.);
#16406=ORIENTED_EDGE('',*,*,#12208,.T.);
#16407=ORIENTED_EDGE('',*,*,#12183,.T.);
#16408=ORIENTED_EDGE('',*,*,#12207,.T.);
#16409=ORIENTED_EDGE('',*,*,#12168,.T.);
#16410=ORIENTED_EDGE('',*,*,#12206,.T.);
#16411=ORIENTED_EDGE('',*,*,#12217,.F.);
#16412=ORIENTED_EDGE('',*,*,#12218,.F.);
#16413=ORIENTED_EDGE('',*,*,#12219,.T.);
#16414=ORIENTED_EDGE('',*,*,#12112,.T.);
#16415=ORIENTED_EDGE('',*,*,#12219,.F.);
#16416=ORIENTED_EDGE('',*,*,#12220,.F.);
#16417=ORIENTED_EDGE('',*,*,#12221,.T.);
#16418=ORIENTED_EDGE('',*,*,#12218,.T.);
#16419=ORIENTED_EDGE('',*,*,#12221,.F.);
#16420=ORIENTED_EDGE('',*,*,#12220,.T.);
#16421=ORIENTED_EDGE('',*,*,#12133,.T.);
#16422=ORIENTED_EDGE('',*,*,#12136,.T.);
#16423=ORIENTED_EDGE('',*,*,#12139,.T.);
#16424=ORIENTED_EDGE('',*,*,#12142,.T.);
#16425=ORIENTED_EDGE('',*,*,#12145,.T.);
#16426=ORIENTED_EDGE('',*,*,#12148,.T.);
#16427=ORIENTED_EDGE('',*,*,#12151,.T.);
#16428=ORIENTED_EDGE('',*,*,#12154,.T.);
#16429=ORIENTED_EDGE('',*,*,#12157,.T.);
#16430=ORIENTED_EDGE('',*,*,#12127,.T.);
#16431=ORIENTED_EDGE('',*,*,#12222,.F.);
#16432=ORIENTED_EDGE('',*,*,#12122,.T.);
#16433=ORIENTED_EDGE('',*,*,#12123,.T.);
#16434=ORIENTED_EDGE('',*,*,#12126,.T.);
#16435=ORIENTED_EDGE('',*,*,#12130,.F.);
#16436=ORIENTED_EDGE('',*,*,#12119,.T.);
#16437=ORIENTED_EDGE('',*,*,#12222,.T.);
#21364=CONICAL_SURFACE('',#23711,1.73,0.785398163397447);
#21365=CONICAL_SURFACE('',#23712,3.45,0.785398163397448);
#21366=CONICAL_SURFACE('',#23715,3.66,0.785398163397449);
#21832=ADVANCED_FACE('',(#3002,#1647),#2003,.F.);
#21833=ADVANCED_FACE('',(#3003),#2481,.T.);
#21834=ADVANCED_FACE('',(#3004,#1648),#2004,.F.);
#21835=ADVANCED_FACE('',(#3005),#2482,.T.);
#21836=ADVANCED_FACE('',(#3006),#2005,.F.);
#21837=ADVANCED_FACE('',(#3007),#2006,.F.);
#21838=ADVANCED_FACE('',(#3008),#2007,.F.);
#21839=ADVANCED_FACE('',(#3009,#1649),#2008,.T.);
#21840=ADVANCED_FACE('',(#3010),#2483,.F.);
#21841=ADVANCED_FACE('',(#3011),#2484,.F.);
#21842=ADVANCED_FACE('',(#3012),#2485,.F.);
#21843=ADVANCED_FACE('',(#3013),#2486,.F.);
#21844=ADVANCED_FACE('',(#3014),#2487,.F.);
#21845=ADVANCED_FACE('',(#3015),#2488,.F.);
#21846=ADVANCED_FACE('',(#3016),#2489,.F.);
#21847=ADVANCED_FACE('',(#3017),#2490,.F.);
#21848=ADVANCED_FACE('',(#3018),#2491,.F.);
#21849=ADVANCED_FACE('',(#3019),#2492,.F.);
#21850=ADVANCED_FACE('',(#3020,#1650),#2009,.F.);
#21851=ADVANCED_FACE('',(#3021),#2493,.F.);
#21852=ADVANCED_FACE('',(#3022,#1651),#2010,.F.);
#21853=ADVANCED_FACE('',(#3023),#2494,.F.);
#21854=ADVANCED_FACE('',(#3024,#1652),#2011,.F.);
#21855=ADVANCED_FACE('',(#3025),#2495,.F.);
#21856=ADVANCED_FACE('',(#3026,#1653),#2012,.F.);
#21857=ADVANCED_FACE('',(#3027),#2496,.F.);
#21858=ADVANCED_FACE('',(#3028,#1654),#2013,.F.);
#21859=ADVANCED_FACE('',(#3029),#2497,.F.);
#21860=ADVANCED_FACE('',(#3030,#1655),#2014,.F.);
#21861=ADVANCED_FACE('',(#3031),#2498,.F.);
#21862=ADVANCED_FACE('',(#3032,#1656),#2015,.F.);
#21863=ADVANCED_FACE('',(#3033),#2499,.F.);
#21864=ADVANCED_FACE('',(#3034,#1657),#2016,.F.);
#21865=ADVANCED_FACE('',(#3035),#2500,.F.);
#21866=ADVANCED_FACE('',(#3036,#1658),#2017,.F.);
#21867=ADVANCED_FACE('',(#3037,#1659),#2018,.T.);
#21868=ADVANCED_FACE('',(#3038),#2501,.F.);
#21869=ADVANCED_FACE('',(#3039),#21364,.F.);
#21870=ADVANCED_FACE('',(#3040),#21365,.T.);
#21871=ADVANCED_FACE('',(#3041),#2502,.T.);
#21872=ADVANCED_FACE('',(#3042),#21366,.T.);
#21873=ADVANCED_FACE('',(#3043,#1660,#1661,#1662,#1663,#1664,#1665,#1666,
#1667,#1668,#1669),#2019,.T.);
#21874=ADVANCED_FACE('',(#3044),#2503,.F.);
#22813=CLOSED_SHELL('',(#21832,#21833,#21834,#21835,#21836,#21837,#21838,
#21839,#21840,#21841,#21842,#21843,#21844,#21845,#21846,#21847,#21848,#21849,
#21850,#21851,#21852,#21853,#21854,#21855,#21856,#21857,#21858,#21859,#21860,
#21861,#21862,#21863,#21864,#21865,#21866,#21867,#21868,#21869,#21870,#21871,
#21872,#21873,#21874));
#23609=AXIS2_PLACEMENT_3D('',#42030,#26638,#26639);
#23610=AXIS2_PLACEMENT_3D('',#42031,#26640,#26641);
#23611=AXIS2_PLACEMENT_3D('',#42033,#26642,#26643);
#23612=AXIS2_PLACEMENT_3D('',#42035,#26644,#26645);
#23613=AXIS2_PLACEMENT_3D('',#42036,#26646,#26647);
#23614=AXIS2_PLACEMENT_3D('',#42038,#26648,#26649);
#23615=AXIS2_PLACEMENT_3D('',#42040,#26651,#26652);
#23616=AXIS2_PLACEMENT_3D('',#42042,#26653,#26654);
#23617=AXIS2_PLACEMENT_3D('',#42043,#26655,#26656);
#23618=AXIS2_PLACEMENT_3D('',#42046,#26658,#26659);
#23619=AXIS2_PLACEMENT_3D('',#42047,#26660,#26661);
#23620=AXIS2_PLACEMENT_3D('',#42056,#26666,#26667);
#23621=AXIS2_PLACEMENT_3D('',#42062,#26671,#26672);
#23622=AXIS2_PLACEMENT_3D('',#42068,#26676,#26677);
#23623=AXIS2_PLACEMENT_3D('',#42070,#26678,#26679);
#23624=AXIS2_PLACEMENT_3D('',#42071,#26680,#26681);
#23625=AXIS2_PLACEMENT_3D('',#42072,#26682,#26683);
#23626=AXIS2_PLACEMENT_3D('',#42074,#26684,#26685);
#23627=AXIS2_PLACEMENT_3D('',#42077,#26687,#26688);
#23628=AXIS2_PLACEMENT_3D('',#42078,#26689,#26690);
#23629=AXIS2_PLACEMENT_3D('',#42080,#26691,#26692);
#23630=AXIS2_PLACEMENT_3D('',#42083,#26694,#26695);
#23631=AXIS2_PLACEMENT_3D('',#42084,#26696,#26697);
#23632=AXIS2_PLACEMENT_3D('',#42086,#26698,#26699);
#23633=AXIS2_PLACEMENT_3D('',#42089,#26701,#26702);
#23634=AXIS2_PLACEMENT_3D('',#42090,#26703,#26704);
#23635=AXIS2_PLACEMENT_3D('',#42092,#26705,#26706);
#23636=AXIS2_PLACEMENT_3D('',#42095,#26708,#26709);
#23637=AXIS2_PLACEMENT_3D('',#42096,#26710,#26711);
#23638=AXIS2_PLACEMENT_3D('',#42098,#26712,#26713);
#23639=AXIS2_PLACEMENT_3D('',#42101,#26715,#26716);
#23640=AXIS2_PLACEMENT_3D('',#42102,#26717,#26718);
#23641=AXIS2_PLACEMENT_3D('',#42104,#26719,#26720);
#23642=AXIS2_PLACEMENT_3D('',#42107,#26722,#26723);
#23643=AXIS2_PLACEMENT_3D('',#42108,#26724,#26725);
#23644=AXIS2_PLACEMENT_3D('',#42110,#26726,#26727);
#23645=AXIS2_PLACEMENT_3D('',#42113,#26729,#26730);
#23646=AXIS2_PLACEMENT_3D('',#42114,#26731,#26732);
#23647=AXIS2_PLACEMENT_3D('',#42116,#26733,#26734);
#23648=AXIS2_PLACEMENT_3D('',#42119,#26736,#26737);
#23649=AXIS2_PLACEMENT_3D('',#42120,#26738,#26739);
#23650=AXIS2_PLACEMENT_3D('',#42122,#26740,#26741);
#23651=AXIS2_PLACEMENT_3D('',#42125,#26743,#26744);
#23652=AXIS2_PLACEMENT_3D('',#42126,#26745,#26746);
#23653=AXIS2_PLACEMENT_3D('',#42136,#26747,#26748);
#23654=AXIS2_PLACEMENT_3D('',#42139,#26750,#26751);
#23655=AXIS2_PLACEMENT_3D('',#42140,#26752,#26753);
#23656=AXIS2_PLACEMENT_3D('',#42141,#26754,#26755);
#23657=AXIS2_PLACEMENT_3D('',#42142,#26756,#26757);
#23658=AXIS2_PLACEMENT_3D('',#42152,#26758,#26759);
#23659=AXIS2_PLACEMENT_3D('',#42155,#26761,#26762);
#23660=AXIS2_PLACEMENT_3D('',#42156,#26763,#26764);
#23661=AXIS2_PLACEMENT_3D('',#42157,#26765,#26766);
#23662=AXIS2_PLACEMENT_3D('',#42158,#26767,#26768);
#23663=AXIS2_PLACEMENT_3D('',#42168,#26769,#26770);
#23664=AXIS2_PLACEMENT_3D('',#42171,#26772,#26773);
#23665=AXIS2_PLACEMENT_3D('',#42172,#26774,#26775);
#23666=AXIS2_PLACEMENT_3D('',#42173,#26776,#26777);
#23667=AXIS2_PLACEMENT_3D('',#42174,#26778,#26779);
#23668=AXIS2_PLACEMENT_3D('',#42184,#26780,#26781);
#23669=AXIS2_PLACEMENT_3D('',#42187,#26783,#26784);
#23670=AXIS2_PLACEMENT_3D('',#42188,#26785,#26786);
#23671=AXIS2_PLACEMENT_3D('',#42189,#26787,#26788);
#23672=AXIS2_PLACEMENT_3D('',#42190,#26789,#26790);
#23673=AXIS2_PLACEMENT_3D('',#42200,#26791,#26792);
#23674=AXIS2_PLACEMENT_3D('',#42203,#26794,#26795);
#23675=AXIS2_PLACEMENT_3D('',#42204,#26796,#26797);
#23676=AXIS2_PLACEMENT_3D('',#42205,#26798,#26799);
#23677=AXIS2_PLACEMENT_3D('',#42206,#26800,#26801);
#23678=AXIS2_PLACEMENT_3D('',#42216,#26802,#26803);
#23679=AXIS2_PLACEMENT_3D('',#42219,#26805,#26806);
#23680=AXIS2_PLACEMENT_3D('',#42220,#26807,#26808);
#23681=AXIS2_PLACEMENT_3D('',#42221,#26809,#26810);
#23682=AXIS2_PLACEMENT_3D('',#42222,#26811,#26812);
#23683=AXIS2_PLACEMENT_3D('',#42232,#26813,#26814);
#23684=AXIS2_PLACEMENT_3D('',#42235,#26816,#26817);
#23685=AXIS2_PLACEMENT_3D('',#42236,#26818,#26819);
#23686=AXIS2_PLACEMENT_3D('',#42237,#26820,#26821);
#23687=AXIS2_PLACEMENT_3D('',#42238,#26822,#26823);
#23688=AXIS2_PLACEMENT_3D('',#42248,#26824,#26825);
#23689=AXIS2_PLACEMENT_3D('',#42251,#26827,#26828);
#23690=AXIS2_PLACEMENT_3D('',#42252,#26829,#26830);
#23691=AXIS2_PLACEMENT_3D('',#42253,#26831,#26832);
#23692=AXIS2_PLACEMENT_3D('',#42254,#26833,#26834);
#23693=AXIS2_PLACEMENT_3D('',#42264,#26835,#26836);
#23694=AXIS2_PLACEMENT_3D('',#42267,#26838,#26839);
#23695=AXIS2_PLACEMENT_3D('',#42268,#26840,#26841);
#23696=AXIS2_PLACEMENT_3D('',#42269,#26842,#26843);
#23697=AXIS2_PLACEMENT_3D('',#42270,#26844,#26845);
#23698=AXIS2_PLACEMENT_3D('',#42271,#26846,#26847);
#23699=AXIS2_PLACEMENT_3D('',#42272,#26848,#26849);
#23700=AXIS2_PLACEMENT_3D('',#42274,#26850,#26851);
#23701=AXIS2_PLACEMENT_3D('',#42275,#26852,#26853);
#23702=AXIS2_PLACEMENT_3D('',#42276,#26854,#26855);
#23703=AXIS2_PLACEMENT_3D('',#42277,#26856,#26857);
#23704=AXIS2_PLACEMENT_3D('',#42278,#26858,#26859);
#23705=AXIS2_PLACEMENT_3D('',#42279,#26860,#26861);
#23706=AXIS2_PLACEMENT_3D('',#42280,#26862,#26863);
#23707=AXIS2_PLACEMENT_3D('',#42281,#26864,#26865);
#23708=AXIS2_PLACEMENT_3D('',#42283,#26866,#26867);
#23709=AXIS2_PLACEMENT_3D('',#42284,#26868,#26869);
#23710=AXIS2_PLACEMENT_3D('',#42287,#26871,#26872);
#23711=AXIS2_PLACEMENT_3D('',#42288,#26873,#26874);
#23712=AXIS2_PLACEMENT_3D('',#42290,#26876,#26877);
#23713=AXIS2_PLACEMENT_3D('',#42292,#26879,#26880);
#23714=AXIS2_PLACEMENT_3D('',#42294,#26881,#26882);
#23715=AXIS2_PLACEMENT_3D('',#42296,#26884,#26885);
#23716=AXIS2_PLACEMENT_3D('',#42298,#26886,#26887);
#23717=AXIS2_PLACEMENT_3D('',#42300,#26889,#26890);
#23718=AXIS2_PLACEMENT_3D('',#42301,#26891,#26892);
#23719=AXIS2_PLACEMENT_3D('',#42302,#26893,#26894);
#26638=DIRECTION('axis',(0.,0.,1.));
#26639=DIRECTION('refdir',(1.,0.,0.));
#26640=DIRECTION('center_axis',(0.,0.,1.));
#26641=DIRECTION('ref_axis',(1.,0.,0.));
#26642=DIRECTION('center_axis',(0.,0.,1.));
#26643=DIRECTION('ref_axis',(1.,0.,0.));
#26644=DIRECTION('center_axis',(0.,0.,1.));
#26645=DIRECTION('ref_axis',(1.,0.,0.));
#26646=DIRECTION('center_axis',(0.,0.,1.));
#26647=DIRECTION('ref_axis',(1.,0.,0.));
#26648=DIRECTION('center_axis',(0.,0.,1.));
#26649=DIRECTION('ref_axis',(1.,0.,0.));
#26650=DIRECTION('',(0.,0.,1.));
#26651=DIRECTION('center_axis',(0.,0.,-1.));
#26652=DIRECTION('ref_axis',(-1.,0.,0.));
#26653=DIRECTION('center_axis',(0.,0.,-1.));
#26654=DIRECTION('ref_axis',(1.,0.,0.));
#26655=DIRECTION('center_axis',(0.,0.,1.));
#26656=DIRECTION('ref_axis',(1.,0.,0.));
#26657=DIRECTION('',(0.,0.,-1.));
#26658=DIRECTION('center_axis',(0.,0.,1.));
#26659=DIRECTION('ref_axis',(1.,0.,0.));
#26660=DIRECTION('center_axis',(0.,1.,0.));
#26661=DIRECTION('ref_axis',(-1.,0.,0.));
#26662=DIRECTION('',(0.,0.,1.));
#26663=DIRECTION('',(-1.,0.,0.));
#26664=DIRECTION('',(0.,0.,1.));
#26665=DIRECTION('',(1.,0.,0.));
#26666=DIRECTION('center_axis',(1.,0.,0.));
#26667=DIRECTION('ref_axis',(0.,1.,0.));
#26668=DIRECTION('',(0.,-1.,0.));
#26669=DIRECTION('',(0.,1.,0.));
#26670=DIRECTION('',(0.,0.,1.));
#26671=DIRECTION('center_axis',(0.,-1.,0.));
#26672=DIRECTION('ref_axis',(1.,0.,0.));
#26673=DIRECTION('',(0.,0.,-1.));
#26674=DIRECTION('',(-1.,0.,0.));
#26675=DIRECTION('',(1.,0.,0.));
#26676=DIRECTION('center_axis',(0.,0.,-1.));
#26677=DIRECTION('ref_axis',(-1.,0.,0.));
#26678=DIRECTION('center_axis',(0.,0.,1.));
#26679=DIRECTION('ref_axis',(1.,0.,0.));
#26680=DIRECTION('center_axis',(0.,0.,1.));
#26681=DIRECTION('ref_axis',(1.,0.,0.));
#26682=DIRECTION('center_axis',(0.,0.,1.));
#26683=DIRECTION('ref_axis',(1.,0.,0.));
#26684=DIRECTION('center_axis',(0.,0.,1.));
#26685=DIRECTION('ref_axis',(1.,0.,0.));
#26686=DIRECTION('',(0.,0.,1.));
#26687=DIRECTION('center_axis',(0.,0.,-1.));
#26688=DIRECTION('ref_axis',(1.,0.,0.));
#26689=DIRECTION('center_axis',(0.,0.,1.));
#26690=DIRECTION('ref_axis',(1.,0.,0.));
#26691=DIRECTION('center_axis',(0.,0.,1.));
#26692=DIRECTION('ref_axis',(1.,0.,0.));
#26693=DIRECTION('',(0.,0.,1.));
#26694=DIRECTION('center_axis',(0.,0.,-1.));
#26695=DIRECTION('ref_axis',(1.,0.,0.));
#26696=DIRECTION('center_axis',(0.,0.,1.));
#26697=DIRECTION('ref_axis',(1.,0.,0.));
#26698=DIRECTION('center_axis',(0.,0.,1.));
#26699=DIRECTION('ref_axis',(1.,0.,0.));
#26700=DIRECTION('',(0.,0.,1.));
#26701=DIRECTION('center_axis',(0.,0.,-1.));
#26702=DIRECTION('ref_axis',(1.,0.,0.));
#26703=DIRECTION('center_axis',(0.,0.,1.));
#26704=DIRECTION('ref_axis',(1.,0.,0.));
#26705=DIRECTION('center_axis',(0.,0.,1.));
#26706=DIRECTION('ref_axis',(1.,0.,0.));
#26707=DIRECTION('',(0.,0.,1.));
#26708=DIRECTION('center_axis',(0.,0.,-1.));
#26709=DIRECTION('ref_axis',(1.,0.,0.));
#26710=DIRECTION('center_axis',(0.,0.,1.));
#26711=DIRECTION('ref_axis',(1.,0.,0.));
#26712=DIRECTION('center_axis',(0.,0.,1.));
#26713=DIRECTION('ref_axis',(1.,0.,0.));
#26714=DIRECTION('',(0.,0.,1.));
#26715=DIRECTION('center_axis',(0.,0.,-1.));
#26716=DIRECTION('ref_axis',(1.,0.,0.));
#26717=DIRECTION('center_axis',(0.,0.,1.));
#26718=DIRECTION('ref_axis',(1.,0.,0.));
#26719=DIRECTION('center_axis',(0.,0.,1.));
#26720=DIRECTION('ref_axis',(1.,0.,0.));
#26721=DIRECTION('',(0.,0.,1.));
#26722=DIRECTION('center_axis',(0.,0.,-1.));
#26723=DIRECTION('ref_axis',(1.,0.,0.));
#26724=DIRECTION('center_axis',(0.,0.,1.));
#26725=DIRECTION('ref_axis',(1.,0.,0.));
#26726=DIRECTION('center_axis',(0.,0.,1.));
#26727=DIRECTION('ref_axis',(1.,0.,0.));
#26728=DIRECTION('',(0.,0.,1.));
#26729=DIRECTION('center_axis',(0.,0.,-1.));
#26730=DIRECTION('ref_axis',(1.,0.,0.));
#26731=DIRECTION('center_axis',(0.,0.,1.));
#26732=DIRECTION('ref_axis',(1.,0.,0.));
#26733=DIRECTION('center_axis',(0.,0.,1.));
#26734=DIRECTION('ref_axis',(1.,0.,0.));
#26735=DIRECTION('',(0.,0.,1.));
#26736=DIRECTION('center_axis',(0.,0.,-1.));
#26737=DIRECTION('ref_axis',(1.,0.,0.));
#26738=DIRECTION('center_axis',(0.,0.,1.));
#26739=DIRECTION('ref_axis',(1.,0.,0.));
#26740=DIRECTION('center_axis',(0.,0.,1.));
#26741=DIRECTION('ref_axis',(1.,0.,0.));
#26742=DIRECTION('',(0.,0.,1.));
#26743=DIRECTION('center_axis',(0.,0.,-1.));
#26744=DIRECTION('ref_axis',(1.,0.,0.));
#26745=DIRECTION('center_axis',(0.,0.,1.));
#26746=DIRECTION('ref_axis',(1.,0.,0.));
#26747=DIRECTION('center_axis',(0.,0.,1.));
#26748=DIRECTION('ref_axis',(1.,0.,0.));
#26749=DIRECTION('',(0.,0.,1.));
#26750=DIRECTION('center_axis',(0.,0.,1.));
#26751=DIRECTION('ref_axis',(1.,0.,0.));
#26752=DIRECTION('center_axis',(0.,0.,1.));
#26753=DIRECTION('ref_axis',(1.,0.,0.));
#26754=DIRECTION('center_axis',(0.,0.,1.));
#26755=DIRECTION('ref_axis',(1.,0.,0.));
#26756=DIRECTION('center_axis',(0.,0.,1.));
#26757=DIRECTION('ref_axis',(1.,0.,0.));
#26758=DIRECTION('center_axis',(0.,0.,1.));
#26759=DIRECTION('ref_axis',(1.,0.,0.));
#26760=DIRECTION('',(0.,0.,1.));
#26761=DIRECTION('center_axis',(0.,0.,1.));
#26762=DIRECTION('ref_axis',(1.,0.,0.));
#26763=DIRECTION('center_axis',(0.,0.,1.));
#26764=DIRECTION('ref_axis',(1.,0.,0.));
#26765=DIRECTION('center_axis',(0.,0.,1.));
#26766=DIRECTION('ref_axis',(1.,0.,0.));
#26767=DIRECTION('center_axis',(0.,0.,1.));
#26768=DIRECTION('ref_axis',(1.,0.,0.));
#26769=DIRECTION('center_axis',(0.,0.,1.));
#26770=DIRECTION('ref_axis',(1.,0.,0.));
#26771=DIRECTION('',(0.,0.,1.));
#26772=DIRECTION('center_axis',(0.,0.,1.));
#26773=DIRECTION('ref_axis',(1.,0.,0.));
#26774=DIRECTION('center_axis',(0.,0.,1.));
#26775=DIRECTION('ref_axis',(1.,0.,0.));
#26776=DIRECTION('center_axis',(0.,0.,1.));
#26777=DIRECTION('ref_axis',(1.,0.,0.));
#26778=DIRECTION('center_axis',(0.,0.,1.));
#26779=DIRECTION('ref_axis',(1.,0.,0.));
#26780=DIRECTION('center_axis',(0.,0.,1.));
#26781=DIRECTION('ref_axis',(1.,0.,0.));
#26782=DIRECTION('',(0.,0.,1.));
#26783=DIRECTION('center_axis',(0.,0.,1.));
#26784=DIRECTION('ref_axis',(1.,0.,0.));
#26785=DIRECTION('center_axis',(0.,0.,1.));
#26786=DIRECTION('ref_axis',(1.,0.,0.));
#26787=DIRECTION('center_axis',(0.,0.,1.));
#26788=DIRECTION('ref_axis',(1.,0.,0.));
#26789=DIRECTION('center_axis',(0.,0.,1.));
#26790=DIRECTION('ref_axis',(1.,0.,0.));
#26791=DIRECTION('center_axis',(0.,0.,1.));
#26792=DIRECTION('ref_axis',(1.,0.,0.));
#26793=DIRECTION('',(0.,0.,1.));
#26794=DIRECTION('center_axis',(0.,0.,1.));
#26795=DIRECTION('ref_axis',(1.,0.,0.));
#26796=DIRECTION('center_axis',(0.,0.,1.));
#26797=DIRECTION('ref_axis',(1.,0.,0.));
#26798=DIRECTION('center_axis',(0.,0.,1.));
#26799=DIRECTION('ref_axis',(1.,0.,0.));
#26800=DIRECTION('center_axis',(0.,0.,1.));
#26801=DIRECTION('ref_axis',(1.,0.,0.));
#26802=DIRECTION('center_axis',(0.,0.,1.));
#26803=DIRECTION('ref_axis',(1.,0.,0.));
#26804=DIRECTION('',(0.,0.,1.));
#26805=DIRECTION('center_axis',(0.,0.,1.));
#26806=DIRECTION('ref_axis',(1.,0.,0.));
#26807=DIRECTION('center_axis',(0.,0.,1.));
#26808=DIRECTION('ref_axis',(1.,0.,0.));
#26809=DIRECTION('center_axis',(0.,0.,1.));
#26810=DIRECTION('ref_axis',(1.,0.,0.));
#26811=DIRECTION('center_axis',(0.,0.,1.));
#26812=DIRECTION('ref_axis',(1.,0.,0.));
#26813=DIRECTION('center_axis',(0.,0.,1.));
#26814=DIRECTION('ref_axis',(1.,0.,0.));
#26815=DIRECTION('',(0.,0.,1.));
#26816=DIRECTION('center_axis',(0.,0.,1.));
#26817=DIRECTION('ref_axis',(1.,0.,0.));
#26818=DIRECTION('center_axis',(0.,0.,1.));
#26819=DIRECTION('ref_axis',(1.,0.,0.));
#26820=DIRECTION('center_axis',(0.,0.,1.));
#26821=DIRECTION('ref_axis',(1.,0.,0.));
#26822=DIRECTION('center_axis',(0.,0.,1.));
#26823=DIRECTION('ref_axis',(1.,0.,0.));
#26824=DIRECTION('center_axis',(0.,0.,1.));
#26825=DIRECTION('ref_axis',(1.,0.,0.));
#26826=DIRECTION('',(0.,0.,1.));
#26827=DIRECTION('center_axis',(0.,0.,1.));
#26828=DIRECTION('ref_axis',(1.,0.,0.));
#26829=DIRECTION('center_axis',(0.,0.,1.));
#26830=DIRECTION('ref_axis',(1.,0.,0.));
#26831=DIRECTION('center_axis',(0.,0.,1.));
#26832=DIRECTION('ref_axis',(1.,0.,0.));
#26833=DIRECTION('center_axis',(0.,0.,1.));
#26834=DIRECTION('ref_axis',(1.,0.,0.));
#26835=DIRECTION('center_axis',(0.,0.,1.));
#26836=DIRECTION('ref_axis',(1.,0.,0.));
#26837=DIRECTION('',(0.,0.,1.));
#26838=DIRECTION('center_axis',(0.,0.,1.));
#26839=DIRECTION('ref_axis',(1.,0.,0.));
#26840=DIRECTION('center_axis',(0.,0.,1.));
#26841=DIRECTION('ref_axis',(1.,0.,0.));
#26842=DIRECTION('center_axis',(0.,0.,1.));
#26843=DIRECTION('ref_axis',(1.,0.,0.));
#26844=DIRECTION('center_axis',(0.,0.,-1.));
#26845=DIRECTION('ref_axis',(-1.,0.,0.));
#26846=DIRECTION('center_axis',(0.,0.,1.));
#26847=DIRECTION('ref_axis',(1.,0.,0.));
#26848=DIRECTION('center_axis',(0.,0.,1.));
#26849=DIRECTION('ref_axis',(1.,0.,0.));
#26850=DIRECTION('center_axis',(0.,0.,1.));
#26851=DIRECTION('ref_axis',(1.,0.,0.));
#26852=DIRECTION('center_axis',(0.,0.,1.));
#26853=DIRECTION('ref_axis',(1.,0.,0.));
#26854=DIRECTION('center_axis',(0.,0.,1.));
#26855=DIRECTION('ref_axis',(1.,0.,0.));
#26856=DIRECTION('center_axis',(0.,0.,1.));
#26857=DIRECTION('ref_axis',(1.,0.,0.));
#26858=DIRECTION('center_axis',(0.,0.,1.));
#26859=DIRECTION('ref_axis',(1.,0.,0.));
#26860=DIRECTION('center_axis',(0.,0.,1.));
#26861=DIRECTION('ref_axis',(1.,0.,0.));
#26862=DIRECTION('center_axis',(0.,0.,1.));
#26863=DIRECTION('ref_axis',(1.,0.,0.));
#26864=DIRECTION('center_axis',(0.,0.,1.));
#26865=DIRECTION('ref_axis',(1.,0.,0.));
#26866=DIRECTION('center_axis',(0.,0.,1.));
#26867=DIRECTION('ref_axis',(1.,0.,0.));
#26868=DIRECTION('center_axis',(0.,0.,1.));
#26869=DIRECTION('ref_axis',(1.,0.,0.));
#26870=DIRECTION('',(0.,0.,-1.));
#26871=DIRECTION('center_axis',(0.,0.,1.));
#26872=DIRECTION('ref_axis',(1.,0.,0.));
#26873=DIRECTION('center_axis',(0.,0.,-1.));
#26874=DIRECTION('ref_axis',(1.,0.,0.));
#26875=DIRECTION('',(-0.707106781186546,-8.65956056235492E-17,-0.707106781186549));
#26876=DIRECTION('center_axis',(0.,0.,1.));
#26877=DIRECTION('ref_axis',(1.,0.,0.));
#26878=DIRECTION('',(0.707106781186548,8.65956056235494E-17,-0.707106781186548));
#26879=DIRECTION('center_axis',(0.,0.,1.));
#26880=DIRECTION('ref_axis',(1.,0.,0.));
#26881=DIRECTION('center_axis',(0.,0.,1.));
#26882=DIRECTION('ref_axis',(1.,0.,0.));
#26883=DIRECTION('',(0.,0.,-1.));
#26884=DIRECTION('center_axis',(0.,0.,-1.));
#26885=DIRECTION('ref_axis',(1.,0.,0.));
#26886=DIRECTION('center_axis',(0.,0.,1.));
#26887=DIRECTION('ref_axis',(1.,0.,0.));
#26888=DIRECTION('',(-0.707106781186548,-8.65956056235494E-17,-0.707106781186547));
#26889=DIRECTION('center_axis',(0.,0.,1.));
#26890=DIRECTION('ref_axis',(1.,0.,0.));
#26891=DIRECTION('center_axis',(0.,0.,1.));
#26892=DIRECTION('ref_axis',(1.,0.,0.));
#26893=DIRECTION('center_axis',(0.,0.,1.));
#26894=DIRECTION('ref_axis',(-1.,-1.22464679914735E-16,0.));
#42030=CARTESIAN_POINT('',(0.,0.,0.));
#42031=CARTESIAN_POINT('Origin',(3.6,0.,-2.4));
#42032=CARTESIAN_POINT('',(-3.7,-4.53119315684521E-16,-2.4));
#42033=CARTESIAN_POINT('Origin',(0.,0.,-2.4));
#42034=CARTESIAN_POINT('',(-3.6,-4.40872847693047E-16,-2.4));
#42035=CARTESIAN_POINT('Origin',(0.,0.,-2.4));
#42036=CARTESIAN_POINT('Origin',(0.,0.,-2.55));
#42037=CARTESIAN_POINT('',(-3.6,-4.40872847693047E-16,-2.7));
#42038=CARTESIAN_POINT('Origin',(0.,0.,-2.7));
#42039=CARTESIAN_POINT('',(-3.6,-4.40872847693047E-16,-2.55));
#42040=CARTESIAN_POINT('Origin',(3.8,0.,-2.7));
#42041=CARTESIAN_POINT('',(-3.7,4.53119315684521E-16,-2.7));
#42042=CARTESIAN_POINT('Origin',(0.,0.,-2.7));
#42043=CARTESIAN_POINT('Origin',(0.,0.,-2.5425));
#42044=CARTESIAN_POINT('',(-3.7,-4.53119315684521E-16,-5.));
#42045=CARTESIAN_POINT('',(-3.7,-4.53119315684521E-16,-2.5425));
#42046=CARTESIAN_POINT('Origin',(0.,0.,-5.));
#42047=CARTESIAN_POINT('Origin',(1.58,0.402,-2.));
#42048=CARTESIAN_POINT('',(1.18570654042221,0.402,-2.));
#42049=CARTESIAN_POINT('',(1.18570654042221,0.402,-0.00499999999999989));
#42050=CARTESIAN_POINT('',(1.18570654042221,0.402,-1.0025));
#42051=CARTESIAN_POINT('',(1.58,0.402,-2.));
#42052=CARTESIAN_POINT('',(1.64,0.402,-2.));
#42053=CARTESIAN_POINT('',(1.58,0.402,-0.00499999999999989));
#42054=CARTESIAN_POINT('',(1.58,0.402,-2.));
#42055=CARTESIAN_POINT('',(1.416,0.402,-0.005));
#42056=CARTESIAN_POINT('Origin',(1.58,-0.402,-2.));
#42057=CARTESIAN_POINT('',(1.58,-0.402,-0.00499999999999989));
#42058=CARTESIAN_POINT('',(1.58,-0.201,-0.005));
#42059=CARTESIAN_POINT('',(1.58,-0.402,-2.));
#42060=CARTESIAN_POINT('',(1.58,-0.201,-2.));
#42061=CARTESIAN_POINT('',(1.58,-0.402,-2.));
#42062=CARTESIAN_POINT('Origin',(1.1,-0.402,-2.));
#42063=CARTESIAN_POINT('',(1.18570654042221,-0.402,-0.00499999999999989));
#42064=CARTESIAN_POINT('',(1.18570654042221,-0.402,-2.));
#42065=CARTESIAN_POINT('',(1.18570654042221,-0.402,-1.0025));
#42066=CARTESIAN_POINT('',(1.176,-0.402,-0.005));
#42067=CARTESIAN_POINT('',(1.4,-0.402,-2.));
#42068=CARTESIAN_POINT('Origin',(1.7,0.,-2.));
#42069=CARTESIAN_POINT('',(-1.7,-2.0818995585505E-16,-2.));
#42070=CARTESIAN_POINT('Origin',(0.,0.,-2.));
#42071=CARTESIAN_POINT('Origin',(0.,0.,-2.));
#42072=CARTESIAN_POINT('Origin',(0.451485261934018,-2.56050015783174,-1.2));
#42073=CARTESIAN_POINT('',(0.101485261934018,-2.56050015783174,-1.2));
#42074=CARTESIAN_POINT('Origin',(0.451485261934018,-2.56050015783174,-1.2));
#42075=CARTESIAN_POINT('',(0.101485261934018,-2.56050015783174,-0.00499999999999989));
#42076=CARTESIAN_POINT('',(0.101485261934018,-2.56050015783174,-1.2));
#42077=CARTESIAN_POINT('Origin',(0.451485261934018,-2.56050015783174,-0.00499999999999989));
#42078=CARTESIAN_POINT('Origin',(-2.44320081404336,-0.889252372646739,-1.2));
#42079=CARTESIAN_POINT('',(-2.79320081404336,-0.889252372646739,-1.2));
#42080=CARTESIAN_POINT('Origin',(-2.44320081404336,-0.889252372646739,-1.2));
#42081=CARTESIAN_POINT('',(-2.79320081404336,-0.889252372646739,-0.00499999999999989));
#42082=CARTESIAN_POINT('',(-2.79320081404336,-0.889252372646739,-1.2));
#42083=CARTESIAN_POINT('Origin',(-2.44320081404336,-0.889252372646739,-0.00499999999999989));
#42084=CARTESIAN_POINT('Origin',(-2.44320081404336,0.889252372646739,-1.2));
#42085=CARTESIAN_POINT('',(-2.79320081404336,0.889252372646739,-1.2));
#42086=CARTESIAN_POINT('Origin',(-2.44320081404336,0.889252372646739,-1.2));
#42087=CARTESIAN_POINT('',(-2.79320081404336,0.889252372646739,-0.00499999999999989));
#42088=CARTESIAN_POINT('',(-2.79320081404336,0.889252372646739,-1.2));
#42089=CARTESIAN_POINT('Origin',(-2.44320081404336,0.889252372646739,-0.00499999999999989));
#42090=CARTESIAN_POINT('Origin',(0.451485261934019,2.56050015783174,-1.2));
#42091=CARTESIAN_POINT('',(0.101485261934019,2.56050015783174,-1.2));
#42092=CARTESIAN_POINT('Origin',(0.451485261934019,2.56050015783174,-1.2));
#42093=CARTESIAN_POINT('',(0.101485261934019,2.56050015783174,-0.00499999999999989));
#42094=CARTESIAN_POINT('',(0.101485261934019,2.56050015783174,-1.2));
#42095=CARTESIAN_POINT('Origin',(0.451485261934019,2.56050015783174,-0.00499999999999989));
#42096=CARTESIAN_POINT('Origin',(1.99171555210934,1.671247785185,-1.2));
#42097=CARTESIAN_POINT('',(1.64171555210934,1.671247785185,-1.2));
#42098=CARTESIAN_POINT('Origin',(1.99171555210934,1.671247785185,-1.2));
#42099=CARTESIAN_POINT('',(1.64171555210934,1.671247785185,-0.00499999999999989));
#42100=CARTESIAN_POINT('',(1.64171555210934,1.671247785185,-1.2));
#42101=CARTESIAN_POINT('Origin',(1.99171555210934,1.671247785185,-0.00499999999999989));
#42102=CARTESIAN_POINT('Origin',(-1.3,2.25166604983954,-1.2));
#42103=CARTESIAN_POINT('',(-1.65,2.25166604983954,-1.2));
#42104=CARTESIAN_POINT('Origin',(-1.3,2.25166604983954,-1.2));
#42105=CARTESIAN_POINT('',(-1.65,2.25166604983954,-0.00499999999999989));
#42106=CARTESIAN_POINT('',(-1.65,2.25166604983954,-1.2));
#42107=CARTESIAN_POINT('Origin',(-1.3,2.25166604983954,-0.00499999999999989));
#42108=CARTESIAN_POINT('Origin',(2.6,0.,-1.2));
#42109=CARTESIAN_POINT('',(2.25,-4.28626379701574E-17,-1.2));
#42110=CARTESIAN_POINT('Origin',(2.6,0.,-1.2));
#42111=CARTESIAN_POINT('',(2.25,4.28626379701574E-17,-0.00499999999999989));
#42112=CARTESIAN_POINT('',(2.25,-4.28626379701574E-17,-1.2));
#42113=CARTESIAN_POINT('Origin',(2.6,0.,-0.00499999999999989));
#42114=CARTESIAN_POINT('Origin',(-1.3,-2.25166604983954,-1.2));
#42115=CARTESIAN_POINT('',(-1.65,-2.25166604983954,-1.2));
#42116=CARTESIAN_POINT('Origin',(-1.3,-2.25166604983954,-1.2));
#42117=CARTESIAN_POINT('',(-1.65,-2.25166604983954,-0.00499999999999989));
#42118=CARTESIAN_POINT('',(-1.65,-2.25166604983954,-1.2));
#42119=CARTESIAN_POINT('Origin',(-1.3,-2.25166604983954,-0.00499999999999989));
#42120=CARTESIAN_POINT('Origin',(1.99171555210934,-1.671247785185,-1.2));
#42121=CARTESIAN_POINT('',(1.64171555210934,-1.671247785185,-1.2));
#42122=CARTESIAN_POINT('Origin',(1.99171555210934,-1.671247785185,-1.2));
#42123=CARTESIAN_POINT('',(1.64171555210934,-1.671247785185,-0.00499999999999989));
#42124=CARTESIAN_POINT('',(1.64171555210934,-1.671247785185,-1.2));
#42125=CARTESIAN_POINT('Origin',(1.99171555210934,-1.671247785185,-0.00499999999999989));
#42126=CARTESIAN_POINT('Origin',(0.451485261934018,-2.56050015783174,-5.5));
#42127=CARTESIAN_POINT('',(0.517772072056189,-3.15783344738108,-5.5));
#42128=CARTESIAN_POINT('',(0.593496052911633,-3.14448126646961,-5.5));
#42129=CARTESIAN_POINT('Ctrl Pts',(0.517772072056188,-3.15783344738107,
-5.5));
#42130=CARTESIAN_POINT('Ctrl Pts',(0.530527217850702,-3.15641799315786,
-5.49933297200685));
#42131=CARTESIAN_POINT('Ctrl Pts',(0.543231868402549,-3.15459414946623,
-5.499));
#42132=CARTESIAN_POINT('Ctrl Pts',(0.568463765021136,-3.15014508531793,
-5.499));
#42133=CARTESIAN_POINT('Ctrl Pts',(0.581026022675185,-3.14751369137377,
-5.49933297200685));
#42134=CARTESIAN_POINT('Ctrl Pts',(0.593496052911633,-3.14448126646961,
-5.5));
#42135=CARTESIAN_POINT('',(-0.149514738065982,-2.56050015783174,-5.5));
#42136=CARTESIAN_POINT('Origin',(0.451485261934018,-2.56050015783174,-5.5));
#42137=CARTESIAN_POINT('',(-0.149514738065982,-2.56050015783174,-1.2));
#42138=CARTESIAN_POINT('',(-0.149514738065982,-2.56050015783174,-5.5));
#42139=CARTESIAN_POINT('Origin',(0.451485261934018,-2.56050015783174,-1.2));
#42140=CARTESIAN_POINT('Origin',(0.451485261934018,-2.56050015783174,-5.5));
#42141=CARTESIAN_POINT('Origin',(0.451485261934018,-2.56050015783174,-1.2));
#42142=CARTESIAN_POINT('Origin',(-2.44320081404336,-0.889252372646739,-5.5));
#42143=CARTESIAN_POINT('',(-3.01994868494276,-1.05825797436754,-5.5));
#42144=CARTESIAN_POINT('',(-2.9936500223803,-1.13051295591977,-5.5));
#42145=CARTESIAN_POINT('Ctrl Pts',(-3.01994868494276,-1.05825797436754,
-5.5));
#42146=CARTESIAN_POINT('Ctrl Pts',(-3.01633982682661,-1.07057354979034,
-5.49933297200685));
#42147=CARTESIAN_POINT('Ctrl Pts',(-3.01233755200259,-1.08276848101971,
-5.499));
#42148=CARTESIAN_POINT('Ctrl Pts',(-3.00357460626879,-1.10684447655122,
-5.499));
#42149=CARTESIAN_POINT('Ctrl Pts',(-2.99880177596235,-1.11875894852114,
-5.49933297200685));
#42150=CARTESIAN_POINT('Ctrl Pts',(-2.9936500223803,-1.13051295591977,-5.5));
#42151=CARTESIAN_POINT('',(-3.04420081404336,-0.889252372646739,-5.5));
#42152=CARTESIAN_POINT('Origin',(-2.44320081404336,-0.889252372646739,-5.5));
#42153=CARTESIAN_POINT('',(-3.04420081404336,-0.889252372646739,-1.2));
#42154=CARTESIAN_POINT('',(-3.04420081404336,-0.889252372646739,-5.5));
#42155=CARTESIAN_POINT('Origin',(-2.44320081404336,-0.889252372646739,-1.2));
#42156=CARTESIAN_POINT('Origin',(-2.44320081404336,-0.889252372646739,-5.5));
#42157=CARTESIAN_POINT('Origin',(-2.44320081404336,-0.889252372646739,-1.2));
#42158=CARTESIAN_POINT('Origin',(-2.44320081404336,0.889252372646739,-5.5));
#42159=CARTESIAN_POINT('',(-2.9936500223803,1.13051295591977,-5.5));
#42160=CARTESIAN_POINT('',(-3.01994868494276,1.05825797436754,-5.5));
#42161=CARTESIAN_POINT('Ctrl Pts',(-2.9936500223803,1.13051295591977,-5.5));
#42162=CARTESIAN_POINT('Ctrl Pts',(-2.99880177596235,1.11875894852114,-5.49933297200685));
#42163=CARTESIAN_POINT('Ctrl Pts',(-3.00357460626879,1.10684447655122,-5.499));
#42164=CARTESIAN_POINT('Ctrl Pts',(-3.01233755200259,1.08276848101971,-5.499));
#42165=CARTESIAN_POINT('Ctrl Pts',(-3.01633982682661,1.07057354979034,-5.49933297200685));
#42166=CARTESIAN_POINT('Ctrl Pts',(-3.01994868494276,1.05825797436754,-5.5));
#42167=CARTESIAN_POINT('',(-3.04420081404336,0.889252372646739,-5.5));
#42168=CARTESIAN_POINT('Origin',(-2.44320081404336,0.889252372646739,-5.5));
#42169=CARTESIAN_POINT('',(-3.04420081404336,0.889252372646739,-1.2));
#42170=CARTESIAN_POINT('',(-3.04420081404336,0.889252372646739,-5.5));
#42171=CARTESIAN_POINT('Origin',(-2.44320081404336,0.889252372646739,-1.2));
#42172=CARTESIAN_POINT('Origin',(-2.44320081404336,0.889252372646739,-5.5));
#42173=CARTESIAN_POINT('Origin',(-2.44320081404336,0.889252372646739,-1.2));
#42174=CARTESIAN_POINT('Origin',(0.451485261934019,2.56050015783174,-5.5));
#42175=CARTESIAN_POINT('',(0.593496052911635,3.14448126646961,-5.5));
#42176=CARTESIAN_POINT('',(0.51777207205619,3.15783344738107,-5.5));
#42177=CARTESIAN_POINT('Ctrl Pts',(0.593496052911635,3.14448126646961,-5.5));
#42178=CARTESIAN_POINT('Ctrl Pts',(0.581026022675186,3.14751369137377,-5.49933297200685));
#42179=CARTESIAN_POINT('Ctrl Pts',(0.568463765021138,3.15014508531793,-5.499));
#42180=CARTESIAN_POINT('Ctrl Pts',(0.543231868402551,3.15459414946623,-5.499));
#42181=CARTESIAN_POINT('Ctrl Pts',(0.530527217850703,3.15641799315786,-5.49933297200685));
#42182=CARTESIAN_POINT('Ctrl Pts',(0.51777207205619,3.15783344738107,-5.5));
#42183=CARTESIAN_POINT('',(-0.149514738065981,2.56050015783174,-5.5));
#42184=CARTESIAN_POINT('Origin',(0.451485261934019,2.56050015783174,-5.5));
#42185=CARTESIAN_POINT('',(-0.149514738065981,2.56050015783174,-1.2));
#42186=CARTESIAN_POINT('',(-0.149514738065981,2.56050015783174,-5.5));
#42187=CARTESIAN_POINT('Origin',(0.451485261934019,2.56050015783174,-1.2));
#42188=CARTESIAN_POINT('Origin',(0.451485261934019,2.56050015783174,-5.5));
#42189=CARTESIAN_POINT('Origin',(0.451485261934019,2.56050015783174,-1.2));
#42190=CARTESIAN_POINT('Origin',(1.99171555210934,1.671247785185,-5.5));
#42191=CARTESIAN_POINT('',(2.47587795032411,2.0273204914613,-5.5));
#42192=CARTESIAN_POINT('',(2.42645263203113,2.08622329210207,-5.5));
#42193=CARTESIAN_POINT('Ctrl Pts',(2.47587795032411,2.0273204914613,-5.5));
#42194=CARTESIAN_POINT('Ctrl Pts',(2.46827455811165,2.03765904463672,-5.49933297200685));
#42195=CARTESIAN_POINT('Ctrl Pts',(2.46034273786624,2.04774967291501,-5.499));
#42196=CARTESIAN_POINT('Ctrl Pts',(2.44387378698146,2.06737660429821,-5.499));
#42197=CARTESIAN_POINT('Ctrl Pts',(2.43531380415142,2.07694014158343,-5.49933297200685));
#42198=CARTESIAN_POINT('Ctrl Pts',(2.42645263203113,2.08622329210207,-5.5));
#42199=CARTESIAN_POINT('',(1.39071555210934,1.671247785185,-5.5));
#42200=CARTESIAN_POINT('Origin',(1.99171555210934,1.671247785185,-5.5));
#42201=CARTESIAN_POINT('',(1.39071555210934,1.671247785185,-1.2));
#42202=CARTESIAN_POINT('',(1.39071555210934,1.671247785185,-5.5));
#42203=CARTESIAN_POINT('Origin',(1.99171555210934,1.671247785185,-1.2));
#42204=CARTESIAN_POINT('Origin',(1.99171555210934,1.671247785185,-5.5));
#42205=CARTESIAN_POINT('Origin',(1.99171555210934,1.671247785185,-1.2));
#42206=CARTESIAN_POINT('Origin',(-1.3,2.25166604983954,-5.5));
#42207=CARTESIAN_POINT('',(-1.5665892436321,2.79030430988024,-5.5));
#42208=CARTESIAN_POINT('',(-1.63317979482944,2.75185823722096,-5.5));
#42209=CARTESIAN_POINT('Ctrl Pts',(-1.5665892436321,2.79030430988024,-5.5));
#42210=CARTESIAN_POINT('Ctrl Pts',(-1.57809104615595,2.78461170119884,-5.49933297200685));
#42211=CARTESIAN_POINT('Ctrl Pts',(-1.58940572124837,2.7785526023377,-5.499));
#42212=CARTESIAN_POINT('Ctrl Pts',(-1.61159427875162,2.76574203269027,-5.499));
#42213=CARTESIAN_POINT('Ctrl Pts',(-1.62249894983562,2.75897278605524,-5.49933297200685));
#42214=CARTESIAN_POINT('Ctrl Pts',(-1.63317979482944,2.75185823722096,-5.5));
#42215=CARTESIAN_POINT('',(-1.901,2.25166604983954,-5.5));
#42216=CARTESIAN_POINT('Origin',(-1.3,2.25166604983954,-5.5));
#42217=CARTESIAN_POINT('',(-1.901,2.25166604983954,-1.2));
#42218=CARTESIAN_POINT('',(-1.901,2.25166604983954,-5.5));
#42219=CARTESIAN_POINT('Origin',(-1.3,2.25166604983954,-1.2));
#42220=CARTESIAN_POINT('Origin',(-1.3,2.25166604983954,-5.5));
#42221=CARTESIAN_POINT('Origin',(-1.3,2.25166604983954,-1.2));
#42222=CARTESIAN_POINT('Origin',(2.6,0.,-5.5));
#42223=CARTESIAN_POINT('',(3.19976903846154,-0.0384460726592727,-5.5));
#42224=CARTESIAN_POINT('',(3.19976903846154,0.0384460726592727,-5.5));
#42225=CARTESIAN_POINT('Ctrl Pts',(3.19976903846154,-0.0384460726592726,
-5.5));
#42226=CARTESIAN_POINT('Ctrl Pts',(3.20058999599157,-0.0256389151436019,
-5.49933297200685));
#42227=CARTESIAN_POINT('Ctrl Pts',(3.201,-0.0128105696474314,-5.499));
#42228=CARTESIAN_POINT('Ctrl Pts',(3.201,0.0128105696474314,-5.499));
#42229=CARTESIAN_POINT('Ctrl Pts',(3.20058999599157,0.0256389151436019,
-5.49933297200685));
#42230=CARTESIAN_POINT('Ctrl Pts',(3.19976903846154,0.0384460726592726,
-5.5));
#42231=CARTESIAN_POINT('',(1.999,-7.36012726287559E-17,-5.5));
#42232=CARTESIAN_POINT('Origin',(2.6,0.,-5.5));
#42233=CARTESIAN_POINT('',(1.999,-7.36012726287559E-17,-1.2));
#42234=CARTESIAN_POINT('',(1.999,-7.36012726287559E-17,-5.5));
#42235=CARTESIAN_POINT('Origin',(2.6,0.,-1.2));
#42236=CARTESIAN_POINT('Origin',(2.6,0.,-5.5));
#42237=CARTESIAN_POINT('Origin',(2.6,0.,-1.2));
#42238=CARTESIAN_POINT('Origin',(-1.3,-2.25166604983954,-5.5));
#42239=CARTESIAN_POINT('',(-1.63317979482944,-2.75185823722096,-5.5));
#42240=CARTESIAN_POINT('',(-1.5665892436321,-2.79030430988023,-5.5));
#42241=CARTESIAN_POINT('Ctrl Pts',(-1.63317979482944,-2.75185823722096,
-5.5));
#42242=CARTESIAN_POINT('Ctrl Pts',(-1.62249894983562,-2.75897278605523,
-5.49933297200685));
#42243=CARTESIAN_POINT('Ctrl Pts',(-1.61159427875163,-2.76574203269027,
-5.499));
#42244=CARTESIAN_POINT('Ctrl Pts',(-1.58940572124838,-2.7785526023377,-5.499));
#42245=CARTESIAN_POINT('Ctrl Pts',(-1.57809104615595,-2.78461170119884,
-5.49933297200685));
#42246=CARTESIAN_POINT('Ctrl Pts',(-1.5665892436321,-2.79030430988023,-5.5));
#42247=CARTESIAN_POINT('',(-1.901,-2.25166604983954,-5.5));
#42248=CARTESIAN_POINT('Origin',(-1.3,-2.25166604983954,-5.5));
#42249=CARTESIAN_POINT('',(-1.901,-2.25166604983954,-1.2));
#42250=CARTESIAN_POINT('',(-1.901,-2.25166604983954,-5.5));
#42251=CARTESIAN_POINT('Origin',(-1.3,-2.25166604983954,-1.2));
#42252=CARTESIAN_POINT('Origin',(-1.3,-2.25166604983954,-5.5));
#42253=CARTESIAN_POINT('Origin',(-1.3,-2.25166604983954,-1.2));
#42254=CARTESIAN_POINT('Origin',(1.99171555210934,-1.671247785185,-5.5));
#42255=CARTESIAN_POINT('',(2.42645263203113,-2.08622329210207,-5.5));
#42256=CARTESIAN_POINT('',(2.47587795032411,-2.02732049146131,-5.5));
#42257=CARTESIAN_POINT('Ctrl Pts',(2.42645263203113,-2.08622329210207,-5.5));
#42258=CARTESIAN_POINT('Ctrl Pts',(2.43531380415142,-2.07694014158343,-5.49933297200685));
#42259=CARTESIAN_POINT('Ctrl Pts',(2.44387378698145,-2.06737660429822,-5.499));
#42260=CARTESIAN_POINT('Ctrl Pts',(2.46034273786624,-2.04774967291501,-5.499));
#42261=CARTESIAN_POINT('Ctrl Pts',(2.46827455811165,-2.03765904463672,-5.49933297200685));
#42262=CARTESIAN_POINT('Ctrl Pts',(2.4758779503241,-2.02732049146131,-5.5));
#42263=CARTESIAN_POINT('',(1.39071555210934,-1.671247785185,-5.5));
#42264=CARTESIAN_POINT('Origin',(1.99171555210934,-1.671247785185,-5.5));
#42265=CARTESIAN_POINT('',(1.39071555210934,-1.671247785185,-1.2));
#42266=CARTESIAN_POINT('',(1.39071555210934,-1.671247785185,-5.5));
#42267=CARTESIAN_POINT('Origin',(1.99171555210934,-1.671247785185,-1.2));
#42268=CARTESIAN_POINT('Origin',(1.99171555210934,-1.671247785185,-5.5));
#42269=CARTESIAN_POINT('Origin',(1.99171555210934,-1.671247785185,-1.2));
#42270=CARTESIAN_POINT('Origin',(3.2,0.,-5.5));
#42271=CARTESIAN_POINT('Origin',(0.,0.,-5.5));
#42272=CARTESIAN_POINT('Origin',(0.,0.,-5.5));
#42273=CARTESIAN_POINT('',(-3.2,-3.91886975727153E-16,-5.5));
#42274=CARTESIAN_POINT('Origin',(0.,0.,-5.5));
#42275=CARTESIAN_POINT('Origin',(0.,0.,-5.5));
#42276=CARTESIAN_POINT('Origin',(0.,0.,-5.5));
#42277=CARTESIAN_POINT('Origin',(0.,0.,-5.5));
#42278=CARTESIAN_POINT('Origin',(0.,0.,-5.5));
#42279=CARTESIAN_POINT('Origin',(0.,0.,-5.5));
#42280=CARTESIAN_POINT('Origin',(0.,0.,-5.5));
#42281=CARTESIAN_POINT('Origin',(0.,0.,-5.5));
#42282=CARTESIAN_POINT('',(-1.76,-2.15537836649934E-16,-5.5));
#42283=CARTESIAN_POINT('Origin',(0.,0.,-5.5));
#42284=CARTESIAN_POINT('Origin',(0.,0.,-3.72));
#42285=CARTESIAN_POINT('',(-1.7,-2.0818995585505E-16,-5.44));
#42286=CARTESIAN_POINT('',(-1.7,-2.0818995585505E-16,-3.72));
#42287=CARTESIAN_POINT('Origin',(0.,0.,-5.44));
#42288=CARTESIAN_POINT('Origin',(0.,0.,-5.47));
#42289=CARTESIAN_POINT('',(-1.73,-2.11863896252492E-16,-5.47));
#42290=CARTESIAN_POINT('Origin',(0.,0.,-5.25));
#42291=CARTESIAN_POINT('',(-3.45,-4.22503145705837E-16,-5.25));
#42292=CARTESIAN_POINT('Origin',(0.,0.,-2.5425));
#42293=CARTESIAN_POINT('',(-3.7,-4.53119315684521E-16,-0.085));
#42294=CARTESIAN_POINT('Origin',(0.,0.,-0.085));
#42295=CARTESIAN_POINT('',(-3.7,-4.53119315684521E-16,-2.5425));
#42296=CARTESIAN_POINT('Origin',(0.,0.,-0.0449999999999999));
#42297=CARTESIAN_POINT('',(-3.62,-4.43322141291342E-16,-0.00499999999999991));
#42298=CARTESIAN_POINT('Origin',(0.,0.,-0.00499999999999989));
#42299=CARTESIAN_POINT('',(-3.66,-4.48220728487931E-16,-0.0449999999999999));
#42300=CARTESIAN_POINT('Origin',(1.252,0.,-0.005));
#42301=CARTESIAN_POINT('Origin',(0.,0.,-0.00499999999999989));
#42302=CARTESIAN_POINT('Origin',(0.,0.,-1.0025));
#59171=UNCERTAINTY_MEASURE_WITH_UNIT(LENGTH_MEASURE(0.001),#59205,
'DISTANCE_ACCURACY_VALUE',
'Maximum model space distance between geometric entities at asserted c
onnectivities');
#59182=UNCERTAINTY_MEASURE_WITH_UNIT(LENGTH_MEASURE(0.001),#59205,
'DISTANCE_ACCURACY_VALUE',
'Maximum model space distance between geometric entities at asserted c
onnectivities');
#59193=(
GEOMETRIC_REPRESENTATION_CONTEXT(3)
GLOBAL_UNCERTAINTY_ASSIGNED_CONTEXT((#59171))
GLOBAL_UNIT_ASSIGNED_CONTEXT((#59205,#59207,#59208))
REPRESENTATION_CONTEXT('','3D')
);
#59204=(
GEOMETRIC_REPRESENTATION_CONTEXT(3)
GLOBAL_UNCERTAINTY_ASSIGNED_CONTEXT((#59182))
GLOBAL_UNIT_ASSIGNED_CONTEXT((#59205,#59207,#59208))
REPRESENTATION_CONTEXT('','3D')
);
#59205=(
LENGTH_UNIT()
NAMED_UNIT(*)
SI_UNIT(.CENTI.,.METRE.)
);
#59207=(
NAMED_UNIT(*)
PLANE_ANGLE_UNIT()
SI_UNIT($,.RADIAN.)
);
#59208=(
NAMED_UNIT(*)
SI_UNIT($,.STERADIAN.)
SOLID_ANGLE_UNIT()
);
#59219=SHAPE_DEFINITION_REPRESENTATION(#59240,#59306);
#59240=PRODUCT_DEFINITION_SHAPE('',$,#59328);
#59306=SHAPE_REPRESENTATION('',(#23609),#59193);
#59317=PRODUCT_DEFINITION_CONTEXT('part definition',#59382,'design');
#59328=PRODUCT_DEFINITION('2026-10-23-00-47-55-837',
'05_Rotary_Cylinder_Block_9xD12',#59349,#59317);
#59349=PRODUCT_DEFINITION_FORMATION('',$,#59394);
#59382=APPLICATION_CONTEXT(
'Core Data for Automotive Mechanical Design Process');
#59383=PRODUCT_CONTEXT('part definition',#59382,'mechanical');
#59394=PRODUCT('2026-10-23-00-47-55-837',
'05_Rotary_Cylinder_Block_9xD12',$,(#59383));
#59559=COLOUR_RGB('Dark Blue',0.08,0.2,0.34);
#59560=FILL_AREA_STYLE_COLOUR('',#59559);
#59561=FILL_AREA_STYLE('',(#59560));
#59562=SURFACE_STYLE_FILL_AREA(#59561);
#59563=SURFACE_SIDE_STYLE('',(#59562));
#59564=SURFACE_STYLE_USAGE(.BOTH.,#59563);
#59565=PRESENTATION_STYLE_ASSIGNMENT((#59564));
ENDSEC;
END-ISO-10303-21;
